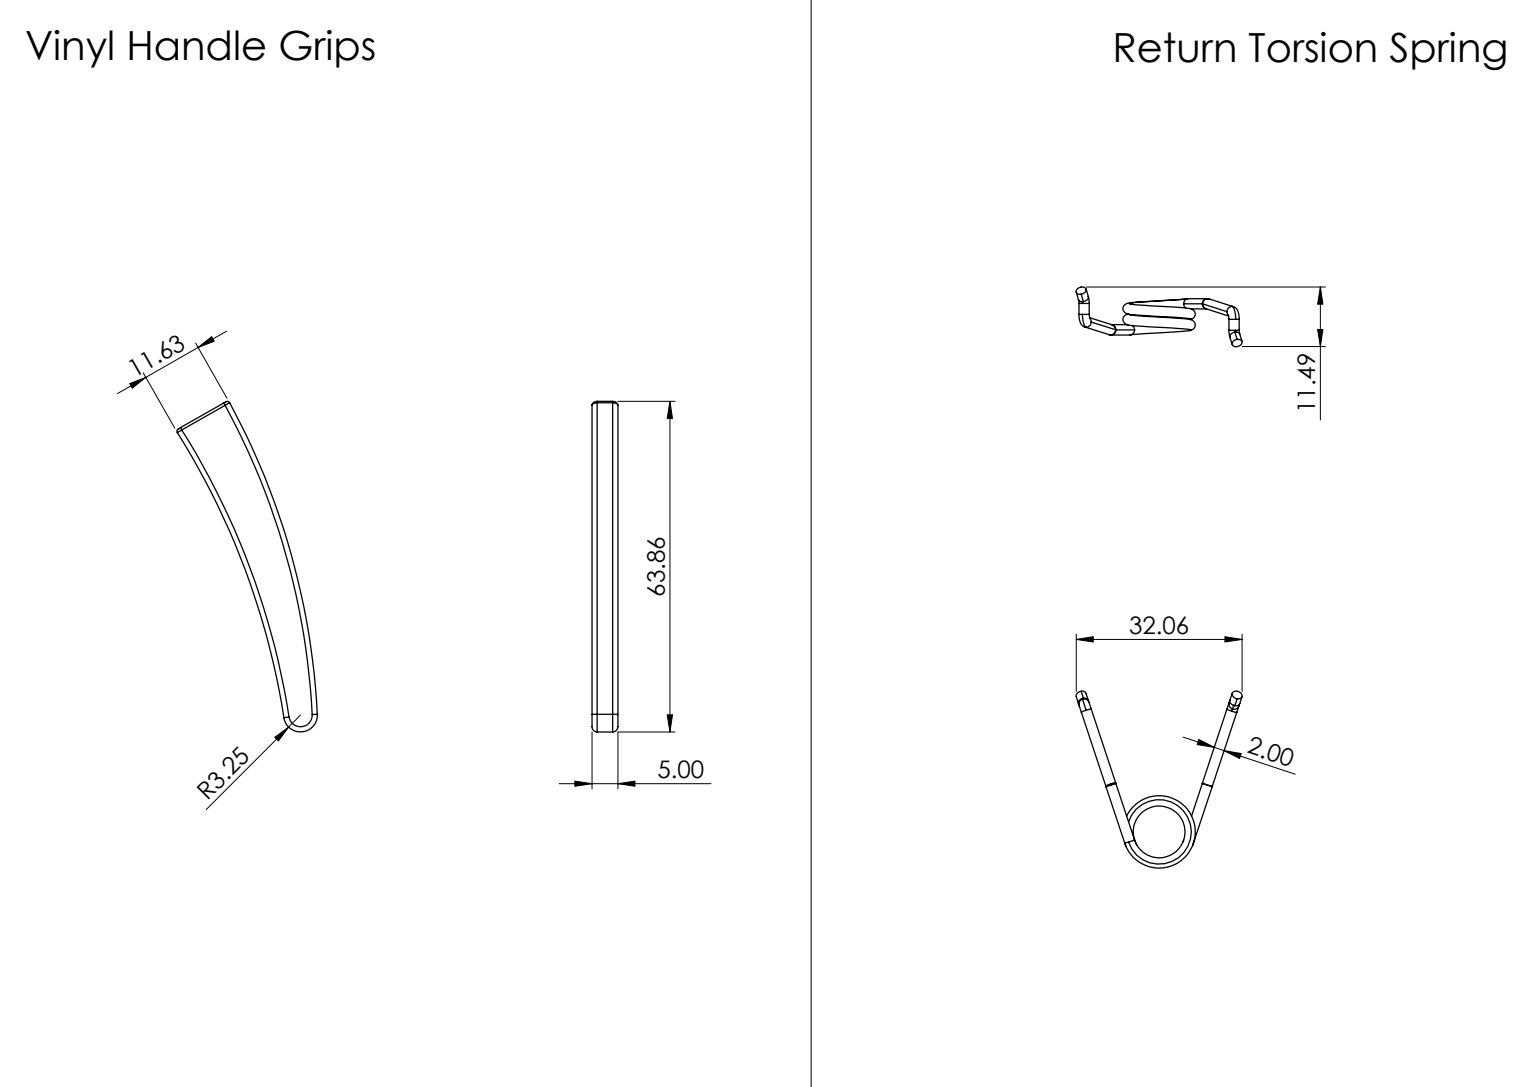
ISO-10303-21;
HEADER;
FILE_DESCRIPTION (('STEP AP214'),
    '1' );
FILE_NAME ('Return Torsion Spring.step',
    '2026-10-09T15:01:35',
    ( '' ),
    ( '' ),
    'SwSTEP 2.0',
    'SolidWorks 2026',
    '' );
FILE_SCHEMA (( 'AUTOMOTIVE_DESIGN' ));
ENDSEC;

DATA;
#6=CARTESIAN_POINT ( 'NONE',  ( -2.243961179877913104, -65.88814609558559710, 1.271710548130833951 ) ) ;
#7=VECTOR ( 'NONE', #4583, 1000.000000000000227 ) ;
#8=CARTESIAN_POINT ( 'NONE',  ( 7.059059989562619819, -58.43975188330606585, -0.3221438859163246460 ) ) ;
#16=CARTESIAN_POINT ( 'NONE',  ( 2.533447467746755333, -55.76293992159236979, -0.1309777151760100067 ) ) ;
#18=FACE_OUTER_BOUND ( 'NONE', #7281, .T. ) ;
#19=CIRCLE ( 'NONE', #5075, 1.000000000000001110 ) ;
#23=LINE ( 'NONE', #5799, #7366 ) ;
#24=AXIS2_PLACEMENT_3D ( 'NONE', #2832, #2306, #6237 ) ;
#29=CARTESIAN_POINT ( 'NONE',  ( -6.272953878096410030, -61.45586155529391448, 1.493064301322690968 ) ) ;
#31=CARTESIAN_POINT ( 'NONE',  ( 1.597826897138040048, -55.24069855439622501, 0.3109211183784004184 ) ) ;
#32=CIRCLE ( 'NONE', #2308, 1.000000000000001110 ) ;
#36=CARTESIAN_POINT ( 'NONE',  ( -15.08175531864075047, -34.71610473016205134, -5.729623873133089518 ) ) ;
#38=EDGE_CURVE ( 'NONE', #489, #1005, #19, .T. ) ;
#39=CARTESIAN_POINT ( 'NONE',  ( 9.311407240687648468, -51.41373841511902043, -1.002481404894999928 ) ) ;
#47=AXIS2_PLACEMENT_3D ( 'NONE', #6946, #1636, #2269 ) ;
#54=CARTESIAN_POINT ( 'NONE',  ( -1.794944750655344867, -54.19869589391355191, -2.224588173883939035 ) ) ;
#57=EDGE_LOOP ( 'NONE', ( #3083, #4276, #3063, #5016, #4331, #6608 ) ) ;
#62=CARTESIAN_POINT ( 'NONE',  ( 3.116905194451685013, -55.41725085606579171, 2.344137946175070653 ) ) ;
#66=ORIENTED_EDGE ( 'NONE', *, *, #4521, .T. ) ;
#67=ORIENTED_EDGE ( 'NONE', *, *, #4872, .T. ) ;
#71=CARTESIAN_POINT ( 'NONE',  ( 1.531562167974070077, -54.12800115838471271, -2.047325108518057935 ) ) ;
#73=CARTESIAN_POINT ( 'NONE',  ( 3.016248221826935083, -64.97666327952782694, -3.135076956698916728 ) ) ;
#78=( NAMED_UNIT ( * ) SI_UNIT ( $, .STERADIAN. ) SOLID_ANGLE_UNIT ( ) );
#80=CARTESIAN_POINT ( 'NONE',  ( 8.409045811045761099, -50.95764513735950629, -2.495037190209991707 ) ) ;
#85=CARTESIAN_POINT ( 'NONE',  ( -4.132930949989339631, -63.16624423302310021, 2.163545901557570428 ) ) ;
#86=DIRECTION ( 'NONE',  ( -0.5224671166576538850, 0.8526594349512809368, 0.000000000000000000 ) ) ;
#87=FACE_OUTER_BOUND ( 'NONE', #3155, .T. ) ;
#94=CARTESIAN_POINT ( 'NONE',  ( -2.961840227416660198, -65.56364223063081909, 1.283932781279834900 ) ) ;
#95=CARTESIAN_POINT ( 'NONE',  ( -1.892846266465454841, -54.28526762408564110, -0.1610563749503846620 ) ) ;
#102=CARTESIAN_POINT ( 'NONE',  ( 2.906897738665179975, -66.25564029441702019, 0.8681355557765302322 ) ) ;
#103=DIRECTION ( 'NONE',  ( 0.2223191033124284066, 0.6712482523644728305, 0.7071067811865467956 ) ) ;
#109=CARTESIAN_POINT ( 'NONE',  ( 5.682346379326408403, -62.38461083188095557, -3.511065069215000278 ) ) ;
#113=CARTESIAN_POINT ( 'NONE',  ( 1.437675307311687245, -54.36893612802973763, 0.01823407963783662405 ) ) ;
#116=CARTESIAN_POINT ( 'NONE',  ( 4.115360779042029904, -63.19255852436059229, -2.695130055691413506 ) ) ;
#121=CARTESIAN_POINT ( 'NONE',  ( 2.653562475325737857, -65.64394347387724338, 0.9832085570212988346 ) ) ;
#123=VERTEX_POINT ( 'NONE', #4619 ) ;
#124=CARTESIAN_POINT ( 'NONE',  ( -5.765066695091211280, -62.35357808832723947, 3.545399627195713332 ) ) ;
#127=CARTESIAN_POINT ( 'NONE',  ( 1.275220786007323914, -54.66846601681689322, 0.1350250863793004130 ) ) ;
#128=CARTESIAN_POINT ( 'NONE',  ( 2.080482015124565098, -66.54183146390657555, -1.221303033644861813 ) ) ;
#129=DIRECTION ( 'NONE',  ( -1.602374898470634869E-16, 1.442524254523139935E-17, 1.000000000000000000 ) ) ;
#135=CARTESIAN_POINT ( 'NONE',  ( -6.814417183322500016, -58.48210382454914935, -0.1019614231452001113 ) ) ;
#144=DIRECTION ( 'NONE',  ( 0.2223157560262044585, -0.6712493609847989262, 0.7071067811865449082 ) ) ;
#146=CIRCLE ( 'NONE', #7235, 1.000000000000000888 ) ;
#149=CARTESIAN_POINT ( 'NONE',  ( -5.163597282883630513, -63.01551968439245144, 3.580859834736030312 ) ) ;
#151=VECTOR ( 'NONE', #4371, 999.9999999999998863 ) ;
#153=CARTESIAN_POINT ( 'NONE',  ( -4.969000869418408683, -63.40403411709974790, -2.714243491562927879 ) ) ;
#154=CARTESIAN_POINT ( 'NONE',  ( -2.104778383727555102, -66.59261038346899397, 1.133408834283370137 ) ) ;
#157=CIRCLE ( 'NONE', #1946, 1.000000000000000444 ) ;
#158=EDGE_LOOP ( 'NONE', ( #2587, #5336, #2767, #4336, #3455, #7221 ) ) ;
#159=PRODUCT_DEFINITION_FORMATION_WITH_SPECIFIED_SOURCE ( 'ANY', '', #255, .NOT_KNOWN. ) ;
#162=EDGE_CURVE ( 'NONE', #6490, #232, #2554, .T. ) ;
#167=CARTESIAN_POINT ( 'NONE',  ( -6.199032880790720235, -61.56120177486793210, 3.556545127952429830 ) ) ;
#170=CARTESIAN_POINT ( 'NONE',  ( 5.465222000274489567, -57.03231251543625291, 0.2812537129946697800 ) ) ;
#177=DIRECTION ( 'NONE',  ( -0.9492883822130750993, 0.3144066910790588865, 0.000000000000000000 ) ) ;
#179=CARTESIAN_POINT ( 'NONE',  ( 5.575556491096470779, -57.10417477796837460, -1.782215851858570010 ) ) ;
#180=CARTESIAN_POINT ( 'NONE',  ( 9.311407240687648468, -51.41373841511900622, -2.502481404895003259 ) ) ;
#188=DIRECTION ( 'NONE',  ( 0.3128416502900965290, -0.9445788350777319931, 0.09950339776592478924 ) ) ;
#189=CARTESIAN_POINT ( 'NONE',  ( -3.569041007005829602, -65.81017109676685095, 3.284668648760890264 ) ) ;
#192=CARTESIAN_POINT ( 'NONE',  ( -2.392055737067099841, -65.19778216667813808, -1.190937291917544050 ) ) ;
#193=CARTESIAN_POINT ( 'NONE',  ( -14.49899450467539985, -35.75040780681265318, -0.4662714048949997969 ) ) ;
#195=CARTESIAN_POINT ( 'NONE',  ( -3.055077159899213690, -65.35589988530520600, -0.7735514844714416194 ) ) ;
#197=CARTESIAN_POINT ( 'NONE',  ( 3.257640280419950241, -66.06664283717124420, -1.252360977842533751 ) ) ;
#203=CARTESIAN_POINT ( 'NONE',  ( -3.235261603508409856, -66.01500717273368934, 1.164464255201294929 ) ) ;
#204=CARTESIAN_POINT ( 'NONE',  ( -5.227302941343250353, -58.92678856866081105, -0.2192372590660296439 ) ) ;
#205=CARTESIAN_POINT ( 'NONE',  ( -6.490403473174280791, -62.28500686936251185, 3.403714661497959870 ) ) ;
#210=VERTEX_POINT ( 'NONE', #2865 ) ;
#214=CARTESIAN_POINT ( 'NONE',  ( 14.18471095241310032, -36.69976849081635351, 0.4975185951050001831 ) ) ;
#215=CARTESIAN_POINT ( 'NONE',  ( -1.756031117750795234, -65.59594772693552045, 1.371125244074580030 ) ) ;
#217=EDGE_CURVE ( 'NONE', #3483, #2618, #2661, .T. ) ;
#224=CARTESIAN_POINT ( 'NONE',  ( -6.308476396955129850, -59.14191327212131455, -0.5142043607924547954 ) ) ;
#226=EDGE_CURVE ( 'NONE', #477, #1089, #6052, .T. ) ;
#228=CARTESIAN_POINT ( 'NONE',  ( -5.725946002089390419, -61.92844332740136792, 1.548851071596535123 ) ) ;
#231=CARTESIAN_POINT ( 'NONE',  ( 2.221695044209367698, -65.89517911169727427, -1.088420971642926727 ) ) ;
#232=VERTEX_POINT ( 'NONE', #3010 ) ;
#239=CARTESIAN_POINT ( 'NONE',  ( -6.429839020462739363, -63.58404662519255623, 2.770540757372710328 ) ) ;
#243=AXIS2_PLACEMENT_3D ( 'NONE', #3684, #2023, #7044 ) ;
#246=CARTESIAN_POINT ( 'NONE',  ( -5.466570931786790766, -63.95713299600960511, -2.842748680216657942 ) ) ;
#247=CARTESIAN_POINT ( 'NONE',  ( 2.831152723192955190, -54.81765481733766876, 0.09675599308719184943 ) ) ;
#255=PRODUCT ( 'Return Torsion Spring', 'Return Torsion Spring', '', ( #964 ) ) ;
#258=CARTESIAN_POINT ( 'NONE',  ( -5.971666637568279867, -56.84728173661435591, 1.574849794282134896 ) ) ;
#262=CARTESIAN_POINT ( 'NONE',  ( 4.897692307440769888, -62.02301377339387756, -1.765793165935516829 ) ) ;
#267=CARTESIAN_POINT ( 'NONE',  ( 3.367951392835606406, -65.15049214652208320, -1.167130348240442927 ) ) ;
#272=DIRECTION ( 'NONE',  ( 0.3128463504745285229, 0.9445772445362839997, 0.09950371902099811039 ) ) ;
#276=CARTESIAN_POINT ( 'NONE',  ( -3.156642594714314853, -54.82761582543010093, 1.871643660998590697 ) ) ;
#278=CARTESIAN_POINT ( 'NONE',  ( -1.626396133375414887, -53.66552156771879112, 1.839959185157149957 ) ) ;
#279=DIRECTION ( 'NONE',  ( 0.000000000000000000, -0.7252570966694442678, 0.6884781359858920258 ) ) ;
#289=CARTESIAN_POINT ( 'NONE',  ( 1.662636012147085118, -65.62619303409478277, -3.045852711070930141 ) ) ;
#290=CARTESIAN_POINT ( 'NONE',  ( 4.774359225188401723, -64.47360709931102463, 0.6998940494460414996 ) ) ;
#292=ORIENTED_EDGE ( 'NONE', *, *, #6726, .T. ) ;
#295=ORIENTED_EDGE ( 'NONE', *, *, #5689, .F. ) ;
#296=DIRECTION ( 'NONE',  ( 0.9492899500389736511, 0.3144019573014823488, 0.000000000000000000 ) ) ;
#300=CARTESIAN_POINT ( 'NONE',  ( 6.696612653858620590, -58.50870383553881737, 0.2496331057155200817 ) ) ;
#303=EDGE_CURVE ( 'NONE', #4768, #4244, #4606, .T. ) ;
#306=CARTESIAN_POINT ( 'NONE',  ( -5.408997660349871062, -62.29959681528816873, 3.625047998704080232 ) ) ;
#309=CARTESIAN_POINT ( 'NONE',  ( -0.5318364440386327274, -66.20751837745356738, -3.028967907328838027 ) ) ;
#311=ORIENTED_EDGE ( 'NONE', *, *, #217, .T. ) ;
#312=CARTESIAN_POINT ( 'NONE',  ( 14.02750760687355935, -37.17441268192290238, 0.4975185951050001831 ) ) ;
#314=DIRECTION ( 'NONE',  ( 0.3128416502900965290, -0.9445788350777319931, 0.09950339776592478924 ) ) ;
#315=DIRECTION ( 'NONE',  ( -0.4328040977884316520, 0.5819352847797604200, 0.6884997728872834788 ) ) ;
#317=CARTESIAN_POINT ( 'NONE',  ( 6.075450823322679383, -63.85990335785957228, 0.5148622082158803570 ) ) ;
#324=CARTESIAN_POINT ( 'NONE',  ( -4.747117373927349782, -63.10583374278928659, -0.4844647803776696016 ) ) ;
#326=CARTESIAN_POINT ( 'NONE',  ( -4.385465831998347497, -64.89496069624793506, 1.250664309176121813 ) ) ;
#327=VERTEX_POINT ( 'NONE', #3117 ) ;
#335=CARTESIAN_POINT ( 'NONE',  ( 1.944327905822930136, -53.75057748617523856, 2.017748614706070143 ) ) ;
#336=ORIENTED_EDGE ( 'NONE', *, *, #6986, .T. ) ;
#338=CARTESIAN_POINT ( 'NONE',  ( -1.512046953658800152, -54.18079592905042574, 1.959428465566195543 ) ) ;
#339=EDGE_CURVE ( 'NONE', #4174, #2620, #4361, .T. ) ;
#350=CARTESIAN_POINT ( 'NONE',  ( 3.592758869166885471, -66.41582265024271692, 0.6922273147611399668 ) ) ;
#354=VERTEX_POINT ( 'NONE', #1399 ) ;
#359=CARTESIAN_POINT ( 'NONE',  ( -5.294444503516980483, -61.70453834742492916, -0.3952116983248150084 ) ) ;
#361=CARTESIAN_POINT ( 'NONE',  ( -6.248181790555211279, -60.49255085186674563, 1.512929826500920338 ) ) ;
#362=CARTESIAN_POINT ( 'NONE',  ( -4.797760869400969241, -62.71499483963494015, 1.636667228454699696 ) ) ;
#367=( NAMED_UNIT ( * ) PLANE_ANGLE_UNIT ( ) SI_UNIT ( $, .RADIAN. ) );
#371=CARTESIAN_POINT ( 'NONE',  ( 6.135463341229070444, -63.36916140199613778, -1.604994752452352014 ) ) ;
#374=ADVANCED_FACE ( 'NONE', ( #1915 ), #2901, .T. ) ;
#377=CARTESIAN_POINT ( 'NONE',  ( 15.08188723176695056, -33.99092340910145538, 5.072392329257909616 ) ) ;
#378=DIRECTION ( 'NONE',  ( 0.000000000000000000, -0.7252570966694443788, 0.6884781359858918037 ) ) ;
#380=VERTEX_POINT ( 'NONE', #6559 ) ;
#382=B_SPLINE_CURVE_WITH_KNOTS ( 'NONE', 3,
 ( #5287, #6445, #2450, #5362, #4685, #5889 ),
 .UNSPECIFIED., .F., .F.,
 ( 4, 2, 4 ),
 ( 0.000000000000000000, 0.5000000000000000000, 1.000000000000000000 ),
 .UNSPECIFIED. ) ;
#388=CARTESIAN_POINT ( 'NONE',  ( -6.381106047699259598, -62.60757382768967716, 3.386766328596300113 ) ) ;
#390=AXIS2_PLACEMENT_3D ( 'NONE', #1613, #3079, #7288 ) ;
#396=CARTESIAN_POINT ( 'NONE',  ( 14.63724902514210058, -34.60816281716094522, 2.969700630898919780 ) ) ;
#400=CARTESIAN_POINT ( 'NONE',  ( -4.470547512179178895, -58.04376326654274720, -1.678768375691622960 ) ) ;
#402=CARTESIAN_POINT ( 'NONE',  ( -4.067320158550557174, -55.70390554630877489, -0.2964418605464455014 ) ) ;
#408=CIRCLE ( 'NONE', #6306, 1.000000000000000888 ) ;
#414=CARTESIAN_POINT ( 'NONE',  ( -3.723298236168965047, -66.76642012610518861, 0.4732191326009700938 ) ) ;
#424=AXIS2_PLACEMENT_3D ( 'NONE', #4211, #6401, #703 ) ;
#425=FACE_OUTER_BOUND ( 'NONE', #7112, .T. ) ;
#426=CARTESIAN_POINT ( 'NONE',  ( -6.269521507055145548, -62.51903585589134593, 1.741451463471350936 ) ) ;
#432=CARTESIAN_POINT ( 'NONE',  ( -1.862703854971429873, -67.54117654042293850, 0.3860096597272351659 ) ) ;
#436=CARTESIAN_POINT ( 'NONE',  ( -2.708443266796834781, -56.15294253968003346, -1.503436295530243827 ) ) ;
#440=EDGE_CURVE ( 'NONE', #477, #6355, #744, .T. ) ;
#441=CARTESIAN_POINT ( 'NONE',  ( 1.159677199572074269, -55.50330010691895666, -1.238196965061255650 ) ) ;
#454=CARTESIAN_POINT ( 'NONE',  ( 1.349182120017575981, -67.40498645023109248, 1.310568389067595207 ) ) ;
#455=DIRECTION ( 'NONE',  ( -0.4328040977884316520, 0.5819352847797604200, 0.6884997728872834788 ) ) ;
#458=LINE ( 'NONE', #3308, #1211 ) ;
#459=CARTESIAN_POINT ( 'NONE',  ( -6.392983792945144295, -62.56006988191466434, 1.848553975009203487 ) ) ;
#465=CARTESIAN_POINT ( 'NONE',  ( 6.751207790105429929, -62.61097121624884210, 0.9581327554396804613 ) ) ;
#469=ADVANCED_FACE ( 'NONE', ( #5653 ), #6728, .T. ) ;
#470=CARTESIAN_POINT ( 'NONE',  ( -1.128062821581302000, -55.49617455686423284, 0.7066123397475153611 ) ) ;
#473=CARTESIAN_POINT ( 'NONE',  ( 1.277257345132870148, -65.35512402512885899, -0.3535023904437397113 ) ) ;
#475=CARTESIAN_POINT ( 'NONE',  ( 4.746441911065370611, -62.01614811949030326, -2.502481404895003259 ) ) ;
#476=CARTESIAN_POINT ( 'NONE',  ( -3.427937952159080037, -54.92350006295870202, -2.312565912944844371 ) ) ;
#477=VERTEX_POINT ( 'NONE', #6809 ) ;
#480=AXIS2_PLACEMENT_3D ( 'NONE', #1466, #4941, #1989 ) ;
#482=EDGE_LOOP ( 'NONE', ( #4891, #695, #2259, #4148, #2799, #2578 ) ) ;
#486=CARTESIAN_POINT ( 'NONE',  ( 3.523276076382420019, -54.00647132653568860, -0.5873174244349146367 ) ) ;
#489=VERTEX_POINT ( 'NONE', #4526 ) ;
#492=CARTESIAN_POINT ( 'NONE',  ( -9.311346830843399758, -51.41373841511900622, 2.533728595105000370 ) ) ;
#493=ADVANCED_FACE ( 'NONE', ( #6254 ), #1091, .T. ) ;
#495=CARTESIAN_POINT ( 'NONE',  ( -5.206993624623629913, -63.95781028998001716, 3.417603084305509853 ) ) ;
#500=CIRCLE ( 'NONE', #2164, 0.9999999999999986677 ) ;
#501=ORIENTED_EDGE ( 'NONE', *, *, #5222, .F. ) ;
#503=CARTESIAN_POINT ( 'NONE',  ( -4.748090069711009775, -62.01667038360579198, 2.533819555318849837 ) ) ;
#505=CARTESIAN_POINT ( 'NONE',  ( -1.424128410011220147, -67.64226375110297340, -1.734372748508781870 ) ) ;
#508=ORIENTED_EDGE ( 'NONE', *, *, #1767, .F. ) ;
#509=CARTESIAN_POINT ( 'NONE',  ( -4.739687333205909958, -61.73825078254577647, 2.268939929871689909 ) ) ;
#510=CARTESIAN_POINT ( 'NONE',  ( 8.362118858474568484, -51.09933172403994917, -2.502481404895003259 ) ) ;
#511=LINE ( 'NONE', #5719, #6770 ) ;
#513=CARTESIAN_POINT ( 'NONE',  ( -5.135436550704829628, -59.04801135763068487, 1.370314102932454814 ) ) ;
#517=CARTESIAN_POINT ( 'NONE',  ( -5.091256589979570535, -61.80182140578926919, 1.697438579844070761 ) ) ;
#519=ORIENTED_EDGE ( 'NONE', *, *, #2113, .F. ) ;
#520=AXIS2_PLACEMENT_3D ( 'NONE', #4684, #6372, #4184 ) ;
#522=CIRCLE ( 'NONE', #1723, 0.9999999999999998890 ) ;
#523=CARTESIAN_POINT ( 'NONE',  ( -13.12502771320784056, -36.71825441132875767, 1.026284428608169819 ) ) ;
#525=CARTESIAN_POINT ( 'NONE',  ( -7.069128816957480410, -61.66762450778810489, 2.866206824378770168 ) ) ;
#538=ORIENTED_EDGE ( 'NONE', *, *, #4985, .F. ) ;
#539=TOROIDAL_SURFACE ( 'NONE', #424, 1.500000000000000000, 1.000000000000000000 ) ;
#544=CARTESIAN_POINT ( 'NONE',  ( 3.523276076382420019, -54.00647132653568860, -0.5873174244349146367 ) ) ;
#545=CARTESIAN_POINT ( 'NONE',  ( -6.643389330756649613, -62.64438243220202196, 2.533637634891150459 ) ) ;
#547=CARTESIAN_POINT ( 'NONE',  ( -4.835761215296770388, -62.04624743670729003, 2.958213919140463055 ) ) ;
#550=CARTESIAN_POINT ( 'NONE',  ( 4.922451174039159660, -61.67826628571419434, -0.7081498598146799273 ) ) ;
#562=CARTESIAN_POINT ( 'NONE',  ( -1.564844514157090138, -53.52797147715784121, 0.2502733031487548443 ) ) ;
#570=ORIENTED_EDGE ( 'NONE', *, *, #4038, .F. ) ;
#571=B_SPLINE_CURVE_WITH_KNOTS ( 'NONE', 3,
 ( #1251, #3568, #5855, #6893, #2994, #3601, #5309, #109, #4035, #643 ),
 .UNSPECIFIED., .F., .F.,
 ( 4, 2, 2, 2, 4 ),
 ( 0.000000000000000000, 0.2500000000000000000, 0.5000000000000000000, 0.7500000000000000000, 1.000000000000000000 ),
 .UNSPECIFIED. ) ;
#574=CARTESIAN_POINT ( 'NONE',  ( -5.480856739662490540, -62.25220485324549458, 1.560007870815685260 ) ) ;
#575=CARTESIAN_POINT ( 'NONE',  ( -1.985532163257450078, -53.63691243282757881, -1.870211432998861945 ) ) ;
#583=CARTESIAN_POINT ( 'NONE',  ( -2.642495264810874822, -65.73545435749777255, -0.8365618114303696728 ) ) ;
#589=CARTESIAN_POINT ( 'NONE',  ( -15.08175531864075047, -33.99084820126180517, -5.041145139047909396 ) ) ;
#591=CARTESIAN_POINT ( 'NONE',  ( -6.240992105565960735, -57.07993508854151798, -2.135104940435555765 ) ) ;
#593=CARTESIAN_POINT ( 'NONE',  ( 5.330483863435800274, -59.34891080545844488, 0.6651839376153853012 ) ) ;
#594=EDGE_LOOP ( 'NONE', ( #6937, #821, #6883, #4560, #734, #2839 ) ) ;
#597=DIRECTION ( 'NONE',  ( -0.08966155106958693943, -0.9959722919136836383, 0.000000000000000000 ) ) ;
#607=DIRECTION ( 'NONE',  ( 0.2223191033124283789, 0.6712482523644727195, 0.7071067811865466846 ) ) ;
#608=CARTESIAN_POINT ( 'NONE',  ( 3.189415849367489564, -54.78201482374456788, -1.959602550130806753 ) ) ;
#616=CARTESIAN_POINT ( 'NONE',  ( -14.63712380658832046, -34.60809039433110001, -2.938452842589635683 ) ) ;
#617=CARTESIAN_POINT ( 'NONE',  ( 5.661089107917369745, -62.15448909529578003, 2.785446686898291002 ) ) ;
#628=AXIS2_PLACEMENT_3D ( 'NONE', #5622, #2168, #455 ) ;
#630=CARTESIAN_POINT ( 'NONE',  ( 1.773380156858839873, -67.30899524596459571, -0.8098396333890448551 ) ) ;
#632=CARTESIAN_POINT ( 'NONE',  ( 2.959376181595404720, -55.87711464508088710, 0.4000749283577051951 ) ) ;
#635=ORIENTED_EDGE ( 'NONE', *, *, #339, .F. ) ;
#636=CIRCLE ( 'NONE', #748, 0.9999999999999984457 ) ;
#643=CARTESIAN_POINT ( 'NONE',  ( 5.463696144088109996, -62.30361170774578028, -3.475027489484119769 ) ) ;
#644=CARTESIAN_POINT ( 'NONE',  ( -5.563801105733269914, -63.69014839564722763, 1.341242183458755344 ) ) ;
#645=CARTESIAN_POINT ( 'NONE',  ( 14.41492992182968003, -36.00466816619485400, 4.365285548071359045 ) ) ;
#648=CARTESIAN_POINT ( 'NONE',  ( 2.466033592522905327, -56.00841680802438560, -1.148886392136307943 ) ) ;
#651=CARTESIAN_POINT ( 'NONE',  ( 14.10571919449219891, -36.93826837078879777, -1.990074380419982969 ) ) ;
#653=CARTESIAN_POINT ( 'NONE',  ( 5.771550998859873438, -61.36048738820532122, 0.6685664931038850511 ) ) ;
#654=CARTESIAN_POINT ( 'NONE',  ( 1.915558458284230214, -54.23376817553720031, 0.07315972318039029587 ) ) ;
#658=CARTESIAN_POINT ( 'NONE',  ( -5.343639688141238686, -62.21333143151184686, 3.460348891136710403 ) ) ;
#662=CARTESIAN_POINT ( 'NONE',  ( 1.919155946380425082, -66.03927477571377835, -1.101811511879709826 ) ) ;
#663=CARTESIAN_POINT ( 'NONE',  ( -2.887726905928315269, -66.20272978495717098, -0.9560320787877147897 ) ) ;
#669=EDGE_CURVE ( 'NONE', #3171, #6921, #5083, .T. ) ;
#672=CARTESIAN_POINT ( 'NONE',  ( -3.268733238405740149, -66.73531384189965365, -2.665188268689791862 ) ) ;
#681=CARTESIAN_POINT ( 'NONE',  ( 5.090297305459900556, -61.99464686763499088, 2.430409751936420282 ) ) ;
#683=CARTESIAN_POINT ( 'NONE',  ( 14.97072768011073940, -34.32654753528365177, 2.597518595105000383 ) ) ;
#685=CARTESIAN_POINT ( 'NONE',  ( 6.202282335592980367, -63.50128988325390367, -3.194577187992014622 ) ) ;
#690=CARTESIAN_POINT ( 'NONE',  ( -5.250750166908019878, -57.72135505925717069, -0.3064819419056146188 ) ) ;
#691=CARTESIAN_POINT ( 'NONE',  ( 1.316624512147740012, -66.75104842734066324, 3.019790780136459851 ) ) ;
#692=CARTESIAN_POINT ( 'NONE',  ( 14.49911764349215915, -35.75048010860329839, 0.4975185951050001831 ) ) ;
#693=ORIENTED_EDGE ( 'NONE', *, *, #5607, .F. ) ;
#695=ORIENTED_EDGE ( 'NONE', *, *, #4767, .T. ) ;
#699=CARTESIAN_POINT ( 'NONE',  ( -6.321361399357500410, -61.94876894069515316, -0.6341497168666246909 ) ) ;
#701=ORIENTED_EDGE ( 'NONE', *, *, #1180, .T. ) ;
#703=DIRECTION ( 'NONE',  ( 0.3144019573014849023, -0.9492899500389726519, 0.000000000000000000 ) ) ;
#705=CARTESIAN_POINT ( 'NONE',  ( -1.512046953658800152, -54.18079592905042574, 1.959428465566195543 ) ) ;
#707=EDGE_CURVE ( 'NONE', #3483, #3171, #4003, .T. ) ;
#708=CARTESIAN_POINT ( 'NONE',  ( -2.678905510920184696, -65.04233304593640241, 0.9295552878624004922 ) ) ;
#711=CARTESIAN_POINT ( 'NONE',  ( 14.49911764349215915, -35.75048010860329839, 0.4975185951050001831 ) ) ;
#712=CARTESIAN_POINT ( 'NONE',  ( -0.07696283880832878455, -66.23396610719073863, -3.055188877874750020 ) ) ;
#713=CARTESIAN_POINT ( 'NONE',  ( -5.316774007586650086, -63.89131393482077925, 1.354123676545745170 ) ) ;
#715=CIRCLE ( 'NONE', #1687, 1.000000000000000444 ) ;
#723=CARTESIAN_POINT ( 'NONE',  ( 1.159215146223531834, -55.24985087088717250, -0.2200125624336850272 ) ) ;
#724=CARTESIAN_POINT ( 'NONE',  ( -6.708998324124310741, -61.63987295270813860, 3.437611327301279385 ) ) ;
#732=CARTESIAN_POINT ( 'NONE',  ( -1.855492712959899926, -67.28785520969887557, -0.6321745227666250022 ) ) ;
#734=ORIENTED_EDGE ( 'NONE', *, *, #3822, .F. ) ;
#737=CARTESIAN_POINT ( 'NONE',  ( -14.81339646197689852, -34.80111785677370051, -2.566271404894997499 ) ) ;
#738=EDGE_CURVE ( 'NONE', #7318, #1826, #636, .T. ) ;
#739=DIRECTION ( 'NONE',  ( 0.3144066910790611624, 0.9492883822130743221, 0.000000000000000000 ) ) ;
#743=AXIS2_PLACEMENT_3D ( 'NONE', #312, #6591, #3835 ) ;
#744=CIRCLE ( 'NONE', #628, 1.000000000000000888 ) ;
#747=CARTESIAN_POINT ( 'NONE',  ( 1.626596344682255113, -54.75750786503496670, 2.255510009909589719 ) ) ;
#748=AXIS2_PLACEMENT_3D ( 'NONE', #2153, #1638, #3968 ) ;
#751=AXIS2_PLACEMENT_3D ( 'NONE', #5959, #3597, #6467 ) ;
#753=CARTESIAN_POINT ( 'NONE',  ( -5.431783234843397423, -58.17252153501718226, -0.3016490821137323142 ) ) ;
#754=CARTESIAN_POINT ( 'NONE',  ( 6.180415987647270626, -62.45112898858806716, 0.6030958204723052551 ) ) ;
#756=ORIENTED_EDGE ( 'NONE', *, *, #1602, .T. ) ;
#764=CARTESIAN_POINT ( 'NONE',  ( -6.097705871868670080, -61.85866295707492668, 3.539665806518350610 ) ) ;
#766=CARTESIAN_POINT ( 'NONE',  ( -2.527830428429834964, -65.26309079616396502, -2.780623214462280668 ) ) ;
#768=CARTESIAN_POINT ( 'NONE',  ( -6.129265975028279634, -62.42766041111902098, -0.6909925287373350766 ) ) ;
#773=ORIENTED_EDGE ( 'NONE', *, *, #2365, .T. ) ;
#777=CARTESIAN_POINT ( 'NONE',  ( 5.248671903609490208, -63.99330799355751509, -3.505550301244489741 ) ) ;
#780=DIRECTION ( 'NONE',  ( 0.2164621326156030423, -0.07169280077033016174, 0.9736551173085935540 ) ) ;
#783=CARTESIAN_POINT ( 'NONE',  ( -6.097705871868670080, -61.85866295707492668, 3.539665806518350610 ) ) ;
#784=ORIENTED_EDGE ( 'NONE', *, *, #6468, .F. ) ;
#785=EDGE_LOOP ( 'NONE', ( #5644, #3488, #7009, #2675, #2047, #4651 ) ) ;
#788=CARTESIAN_POINT ( 'NONE',  ( 4.977719985769329725, -63.63849604921595216, 2.874328699340139792 ) ) ;
#789=CARTESIAN_POINT ( 'NONE',  ( 9.311407240687648468, -51.41373841511902043, -1.002481404894999928 ) ) ;
#791=CARTESIAN_POINT ( 'NONE',  ( 4.372548960228861858, -64.23807538291029573, -1.245661913065559734 ) ) ;
#798=CARTESIAN_POINT ( 'NONE',  ( 5.661113010068490325, -57.37064013373739613, 2.401523511004880262 ) ) ;
#799=FACE_OUTER_BOUND ( 'NONE', #1045, .T. ) ;
#801=ORIENTED_EDGE ( 'NONE', *, *, #2322, .T. ) ;
#805=CARTESIAN_POINT ( 'NONE',  ( 9.358334193258830425, -51.27205182843857045, -2.495037190209991707 ) ) ;
#806=DIRECTION ( 'NONE',  ( -0.3144066910790599412, -0.9492883822130747662, 0.000000000000000000 ) ) ;
#807=CARTESIAN_POINT ( 'NONE',  ( 2.440761905804889942, -65.30842328614467363, 1.105894752426585415 ) ) ;
#808=CARTESIAN_POINT ( 'NONE',  ( -5.904042796847299712, -62.42803713013675093, 3.506543003539000392 ) ) ;
#817=CARTESIAN_POINT ( 'NONE',  ( -0.9970853242166300978, -65.67144495878099519, -1.280490079922569802 ) ) ;
#820=CARTESIAN_POINT ( 'NONE',  ( 4.754243898017194603, -57.04914850836969009, -1.691473023288849742 ) ) ;
#821=ORIENTED_EDGE ( 'NONE', *, *, #4240, .T. ) ;
#825=DIRECTION ( 'NONE',  ( 0.1860016876085203719, -0.1636620475539280195, 0.9688230521603200529 ) ) ;
#828=CARTESIAN_POINT ( 'NONE',  ( -1.974098099753330171, -66.57628266072889289, 3.196874607719439876 ) ) ;
#829=CARTESIAN_POINT ( 'NONE',  ( -3.508682979600159957, -66.46637211483655960, 1.044995729122755179 ) ) ;
#833=AXIS2_PLACEMENT_3D ( 'NONE', #2348, #5745, #4043 ) ;
#834=CARTESIAN_POINT ( 'NONE',  ( 9.311407240687648468, -51.41373841511902043, -3.502481404894999706 ) ) ;
#838=CARTESIAN_POINT ( 'NONE',  ( 5.253257825778660184, -59.02147093648149223, -1.455491405082765866 ) ) ;
#839=CARTESIAN_POINT ( 'NONE',  ( 6.214916356356757099, -59.39665835591213749, 2.509282487442340948 ) ) ;
#850=CARTESIAN_POINT ( 'NONE',  ( 3.592758869166885471, -66.41582265024271692, 0.6922273147611399668 ) ) ;
#854=CARTESIAN_POINT ( 'NONE',  ( 14.63724902514210058, -36.05867701049984930, 4.346656902870709160 ) ) ;
#855=CARTESIAN_POINT ( 'NONE',  ( 5.175864525269250116, -61.68163375030346174, 0.3100344153189201202 ) ) ;
#861=CARTESIAN_POINT ( 'NONE',  ( -3.816438721764812136, -64.79865757078124489, -2.819062171272241901 ) ) ;
#865=AXIS2_PLACEMENT_3D ( 'NONE', #7223, #2593, #904 ) ;
#866=CARTESIAN_POINT ( 'NONE',  ( -14.49899450467539985, -35.75040780681265318, -2.566271404894997499 ) ) ;
#870=CARTESIAN_POINT ( 'NONE',  ( -5.628700163094269016, -63.23550210468251009, 3.461537593744290042 ) ) ;
#873=CARTESIAN_POINT ( 'NONE',  ( 6.131131505788760094, -57.13037711201883440, 2.282642250695309905 ) ) ;
#879=ADVANCED_FACE ( 'NONE', ( #799 ), #2886, .T. ) ;
#880=AXIS2_PLACEMENT_3D ( 'NONE', #4624, #4579, #3475 ) ;
#885=CARTESIAN_POINT ( 'NONE',  ( 4.826828241146579934, -57.92957641372471755, 0.5758163846279100717 ) ) ;
#887=CARTESIAN_POINT ( 'NONE',  ( -5.586110484983932700, -63.35381962756557783, 1.355548068171432252 ) ) ;
#898=CARTESIAN_POINT ( 'NONE',  ( 5.267626090836840191, -63.86700364562991439, -1.442031773567929775 ) ) ;
#903=ADVANCED_FACE ( 'NONE', ( #1173 ), #6519, .T. ) ;
#904=DIRECTION ( 'NONE',  ( -0.2163384215910431896, -0.07165063022625259292, 0.9736857165079894072 ) ) ;
#905=CARTESIAN_POINT ( 'NONE',  ( -3.569041007005829602, -65.81017109676685095, 3.284668648760890264 ) ) ;
#906=ORIENTED_EDGE ( 'NONE', *, *, #7286, .F. ) ;
#907=CARTESIAN_POINT ( 'NONE',  ( -6.643389330756649613, -62.64438243220202196, 2.533637634891150459 ) ) ;
#914=CARTESIAN_POINT ( 'NONE',  ( 5.416018991692120643, -63.93240027730202968, 2.754852738177090643 ) ) ;
#915=CARTESIAN_POINT ( 'NONE',  ( 6.647873823884112632, -62.63640551056316497, -2.279271695592409497 ) ) ;
#916=CARTESIAN_POINT ( 'NONE',  ( 6.663059173928499668, -62.48704134639812935, 2.547684199221960100 ) ) ;
#923=CARTESIAN_POINT ( 'NONE',  ( 4.756074659365879143, -62.80135681555328375, -3.311393743080873975 ) ) ;
#926=CARTESIAN_POINT ( 'NONE',  ( -5.894573565049844532, -58.07158296836707478, 1.644009501509583027 ) ) ;
#934=CARTESIAN_POINT ( 'NONE',  ( -1.206827191127304078, -66.77204028133226643, -1.044217440639481742 ) ) ;
#940=CARTESIAN_POINT ( 'NONE',  ( -1.095027572700850049, -66.25608112803911354, -0.9253912358714898589 ) ) ;
#943=EDGE_CURVE ( 'NONE', #2698, #3646, #2185, .T. ) ;
#944=CARTESIAN_POINT ( 'NONE',  ( -5.667613743078470101, -62.32074054030601928, 1.527775587545428193 ) ) ;
#946=CARTESIAN_POINT ( 'NONE',  ( 9.358334193258830425, -51.27205182843857045, -2.495037190209989930 ) ) ;
#948=CARTESIAN_POINT ( 'NONE',  ( 6.319659661046010513, -62.49917928162491876, -1.706589513406323366 ) ) ;
#949=CARTESIAN_POINT ( 'NONE',  ( -1.678659834933539985, -53.30027862203323252, 1.268182062803870247 ) ) ;
#954=CARTESIAN_POINT ( 'NONE',  ( 13.49911764349216092, -35.75048010860329839, 0.4975185951050001831 ) ) ;
#957=CARTESIAN_POINT ( 'NONE',  ( -4.248468832057555211, -63.21868707083201855, -2.033638508047526550 ) ) ;
#959=CARTESIAN_POINT ( 'NONE',  ( 6.164870568366772829, -59.43741054342344654, 0.4113734782956702252 ) ) ;
#964=PRODUCT_CONTEXT ( 'NONE', #2544, 'mechanical' ) ;
#969=CARTESIAN_POINT ( 'NONE',  ( -6.490403473174280791, -62.28500686936251185, 3.403714661497959870 ) ) ;
#973=CARTESIAN_POINT ( 'NONE',  ( 6.285636693253979779, -59.03245517747429716, 2.489777307435960374 ) ) ;
#977=ORIENTED_EDGE ( 'NONE', *, *, #5252, .T. ) ;
#982=LINE ( 'NONE', #1590, #1137 ) ;
#983=DIRECTION ( 'NONE',  ( -0.9492899500389727629, -0.3144019573014849023, 0.000000000000000000 ) ) ;
#984=CARTESIAN_POINT ( 'NONE',  ( 1.349182120017575981, -67.40498645023109248, 1.310568389067595207 ) ) ;
#985=DIRECTION ( 'NONE',  ( 0.1860016876085203441, -0.1636620475539279917, 0.9688230521603200529 ) ) ;
#986=CIRCLE ( 'NONE', #390, 0.9999999999999998890 ) ;
#994=VECTOR ( 'NONE', #5299, 1000.000000000000114 ) ;
#995=DIRECTION ( 'NONE',  ( 0.3144066910790613845, 0.9492883822130742111, 0.000000000000000000 ) ) ;
#996=CARTESIAN_POINT ( 'NONE',  ( -1.630661209647960019, -65.50972637651682362, 2.960670344429949807 ) ) ;
#999=CARTESIAN_POINT ( 'NONE',  ( -4.429163702585058537, -56.03682623248362660, -0.3226722266289872576 ) ) ;
#1001=CARTESIAN_POINT ( 'NONE',  ( 5.674632694949170109, -63.26545500802649258, -3.549449971387770297 ) ) ;
#1005=VERTEX_POINT ( 'NONE', #3490 ) ;
#1010=DIRECTION ( 'NONE',  ( 0.3144066910790610514, 0.9492883822130744331, 0.000000000000000000 ) ) ;
#1013=CARTESIAN_POINT ( 'NONE',  ( -6.126235009943979293, -64.48141016635396738, -1.469515951087519978 ) ) ;
#1018=DIRECTION ( 'NONE',  ( 0.3144019573014853464, -0.9492899500389726519, -7.355227538141627568E-16 ) ) ;
#1019=CARTESIAN_POINT ( 'NONE',  ( 5.929218414971320072, -62.35084102844776055, -1.530333388185332932 ) ) ;
#1028=DIRECTION ( 'NONE',  ( 0.2223157560262043198, -0.6712493609847984821, 0.7071067811865453523 ) ) ;
#1030=CARTESIAN_POINT ( 'NONE',  ( 4.128395891713080523, -66.51223636356003510, -1.999098658498605019 ) ) ;
#1033=VERTEX_POINT ( 'NONE', #36 ) ;
#1035=CARTESIAN_POINT ( 'NONE',  ( -4.410792138572509735, -62.95272468751611683, 0.08690264739508006542 ) ) ;
#1038=CARTESIAN_POINT ( 'NONE',  ( -4.317466541193835106, -57.77653723152862142, 0.4415034884863752729 ) ) ;
#1041=CARTESIAN_POINT ( 'NONE',  ( -0.4891006619385195320, -66.67017596358577691, -1.083201131225852265 ) ) ;
#1043=EDGE_CURVE ( 'NONE', #1750, #4040, #3536, .T. ) ;
#1045=EDGE_LOOP ( 'NONE', ( #4028, #1415, #2287, #784, #2380, #4918 ) ) ;
#1049=DIRECTION ( 'NONE',  ( -1.602374898470634869E-16, 1.442524254523139935E-17, 1.000000000000000000 ) ) ;
#1051=CARTESIAN_POINT ( 'NONE',  ( -5.957512881900739465, -64.40555820178136059, 2.727170671215090270 ) ) ;
#1057=CARTESIAN_POINT ( 'NONE',  ( -6.308476396955129850, -59.14191327212131455, -0.5142043607924547954 ) ) ;
#1066=CARTESIAN_POINT ( 'NONE',  ( 7.124841322228030904, -62.19900605811294980, -0.1440571144897197509 ) ) ;
#1070=CARTESIAN_POINT ( 'NONE',  ( 4.447965418036755381, -62.61493371638615457, -2.739923498411994451 ) ) ;
#1075=CARTESIAN_POINT ( 'NONE',  ( -9.358272925367041140, -51.27205205187813419, 2.526284428608170263 ) ) ;
#1076=CARTESIAN_POINT ( 'NONE',  ( -5.318175601589866908, -63.71090186687732171, -0.7685412544916830901 ) ) ;
#1077=CARTESIAN_POINT ( 'NONE',  ( -6.338727533122220592, -59.01378846946391832, -2.577673957235475211 ) ) ;
#1080=ORIENTED_EDGE ( 'NONE', *, *, #1641, .T. ) ;
#1088=CARTESIAN_POINT ( 'NONE',  ( -3.941959611298590183, -54.25574829393653431, -0.9393447306324897994 ) ) ;
#1089=VERTEX_POINT ( 'NONE', #737 ) ;
#1091=CYLINDRICAL_SURFACE ( 'NONE', #6752, 0.9999999999999988898 ) ;
#1100=CIRCLE ( 'NONE', #3980, 0.9999999999999986677 ) ;
#1104=CARTESIAN_POINT ( 'NONE',  ( -15.08175531864075047, -33.26559167236155190, -4.352666404962730162 ) ) ;
#1105=CARTESIAN_POINT ( 'NONE',  ( -6.238287558858839787, -63.42668406018486849, 1.752565146537014895 ) ) ;
#1108=CARTESIAN_POINT ( 'NONE',  ( -9.311346830843410416, -51.41373841511900622, 1.033728595105000148 ) ) ;
#1109=CARTESIAN_POINT ( 'NONE',  ( -4.317466541193835106, -57.77653723152862142, 0.4415034884863752729 ) ) ;
#1113=CARTESIAN_POINT ( 'NONE',  ( -1.005393588828258133, -65.41824993351924888, -2.298700180912566449 ) ) ;
#1116=CARTESIAN_POINT ( 'NONE',  ( -6.227481695512121718, -59.47789623974718864, -0.5324849168858507564 ) ) ;
#1127=CARTESIAN_POINT ( 'NONE',  ( -8.362056880804429326, -51.09933645781752887, 2.533728595105000370 ) ) ;
#1128=CARTESIAN_POINT ( 'NONE',  ( -4.101849953070630050, -66.53066707031882743, 2.593177719986650143 ) ) ;
#1130=CIRCLE ( 'NONE', #3756, 0.5000000000000066613 ) ;
#1132=EDGE_CURVE ( 'NONE', #489, #4174, #1353, .T. ) ;
#1137=VECTOR ( 'NONE', #4984, 999.9999999999998863 ) ;
#1151=CARTESIAN_POINT ( 'NONE',  ( -1.432436674628349893, -67.38906872584260555, -2.752582849501530760 ) ) ;
#1158=CARTESIAN_POINT ( 'NONE',  ( 2.753836159791509974, -65.67748394244114252, 3.050484385245309849 ) ) ;
#1160=CARTESIAN_POINT ( 'NONE',  ( -4.053309352542619592, -65.19933310964161421, -0.8734501311131982471 ) ) ;
#1167=CARTESIAN_POINT ( 'NONE',  ( -1.985532163257450078, -53.63691243282757881, -1.870211432998861945 ) ) ;
#1169=CARTESIAN_POINT ( 'NONE',  ( 5.271413390890690387, -61.79997272665566044, -1.279516964844005900 ) ) ;
#1172=FILL_AREA_STYLE_COLOUR ( '', #4123 ) ;
#1173=FACE_OUTER_BOUND ( 'NONE', #4086, .T. ) ;
#1178=CARTESIAN_POINT ( 'NONE',  ( 10.30762257547189975, -51.58645851951763461, -2.495037190209991707 ) ) ;
#1180=EDGE_CURVE ( 'NONE', #1972, #123, #157, .T. ) ;
#1184=CARTESIAN_POINT ( 'NONE',  ( -5.205673437485017097, -63.09603712129732855, 1.507649522180431800 ) ) ;
#1185=CARTESIAN_POINT ( 'NONE',  ( 5.396949887678069935, -64.06165292293543700, 0.6913201402231599069 ) ) ;
#1187=EDGE_LOOP ( 'NONE', ( #5457, #3397, #3061, #6621, #1235 ) ) ;
#1188=CARTESIAN_POINT ( 'NONE',  ( -5.011296251047005157, -62.10358530323204462, 3.211213581958491492 ) ) ;
#1193=CARTESIAN_POINT ( 'NONE',  ( -5.689067437457130616, -61.48253059702771850, 3.675478928603590489 ) ) ;
#1194=DIRECTION ( 'NONE',  ( -0.2467992669038191478, 0.02032136184815930280, 0.9688535307818069153 ) ) ;
#1195=DIRECTION ( 'NONE',  ( 0.2223157560262044585, -0.6712493609847989262, 0.7071067811865449082 ) ) ;
#1202=CARTESIAN_POINT ( 'NONE',  ( -2.104778383727555102, -66.59261038346899397, 1.133408834283370137 ) ) ;
#1204=CARTESIAN_POINT ( 'NONE',  ( 2.734303695691099989, -65.14978033110251943, -1.014598242344157963 ) ) ;
#1205=B_SPLINE_CURVE_WITH_KNOTS ( 'NONE', 3,
 ( #5469, #3072, #7099, #5994, #5388, #2513, #4820, #4251, #4524, #1684 ),
 .UNSPECIFIED., .F., .F.,
 ( 4, 2, 2, 2, 4 ),
 ( 0.000000000000000000, 0.2500000000000002776, 0.5000000000000002220, 0.7500000000000001110, 1.000000000000000000 ),
 .UNSPECIFIED. ) ;
#1211=VECTOR ( 'NONE', #5626, 1000.000000000000114 ) ;
#1213=CARTESIAN_POINT ( 'NONE',  ( 3.403992074353090036, -54.97443010399496899, 2.224669212202579960 ) ) ;
#1219=CARTESIAN_POINT ( 'NONE',  ( 15.49911764349215026, -35.75048010860329839, 0.4975185951050001831 ) ) ;
#1220=CARTESIAN_POINT ( 'NONE',  ( 4.719984496330532409, -63.87667799492090381, 0.8260579302787993683 ) ) ;
#1221=CIRCLE ( 'NONE', #5427, 1.000000000000001110 ) ;
#1225=CARTESIAN_POINT ( 'NONE',  ( -5.078718092191791378, -62.12561931644285806, 3.276649263749329855 ) ) ;
#1227=CARTESIAN_POINT ( 'NONE',  ( -10.30756287540601868, -51.58645400917961865, 2.526284428608170263 ) ) ;
#1228=CARTESIAN_POINT ( 'NONE',  ( -1.799724466760814989, -66.07795133246216324, 3.315732812615050484 ) ) ;
#1229=CARTESIAN_POINT ( 'NONE',  ( -6.308476396955129850, -59.14191327212131455, -0.5142043607924547954 ) ) ;
#1235=ORIENTED_EDGE ( 'NONE', *, *, #2956, .F. ) ;
#1238=CIRCLE ( 'NONE', #2899, 1.000000000000001776 ) ;
#1239=AXIS2_PLACEMENT_3D ( 'NONE', #1108, #1751, #5323 ) ;
#1240=CARTESIAN_POINT ( 'NONE',  ( -3.381846796090564933, -54.21055914560344746, 0.1632119451740500493 ) ) ;
#1241=DIRECTION ( 'NONE',  ( 0.3144019573014849023, -0.9492899500389727629, 0.000000000000000000 ) ) ;
#1249=CARTESIAN_POINT ( 'NONE',  ( -14.81339646197689852, -34.80111785677370051, -0.4662714048949997969 ) ) ;
#1251=CARTESIAN_POINT ( 'NONE',  ( 6.643375263299909683, -62.64442119333418901, -2.502572238011808281 ) ) ;
#1254=CIRCLE ( 'NONE', #6772, 1.000000000000001110 ) ;
#1255=CARTESIAN_POINT ( 'NONE',  ( 1.080279179814437773, -65.65553934942860792, 2.784998920779040432 ) ) ;
#1258=DIRECTION ( 'NONE',  ( 2.290931512739800066E-16, 1.403768413105889815E-16, 1.000000000000000000 ) ) ;
#1260=EDGE_CURVE ( 'NONE', #327, #6872, #1366, .T. ) ;
#1262=DIRECTION ( 'NONE',  ( 0.000000000000000000, -0.7252565289002705917, -0.6884787340851793447 ) ) ;
#1263=AXIS2_PLACEMENT_3D ( 'NONE', #2069, #6089, #3989 ) ;
#1270=CARTESIAN_POINT ( 'NONE',  ( -2.889418079045375176, -55.97554976774797098, -0.4852521485111498389 ) ) ;
#1271=CARTESIAN_POINT ( 'NONE',  ( -6.239404450008960268, -62.05055862403510503, 1.429382062327010150 ) ) ;
#1282=CARTESIAN_POINT ( 'NONE',  ( -6.079305786110669629, -62.05959118544440400, 1.459294228111509995 ) ) ;
#1290=CARTESIAN_POINT ( 'NONE',  ( -4.721082446365287844, -64.53544812894149629, 1.276903664564835283 ) ) ;
#1291=CARTESIAN_POINT ( 'NONE',  ( -2.437747074861595031, -55.99259917890189797, 0.6173017669495700632 ) ) ;
#1294=CARTESIAN_POINT ( 'NONE',  ( -4.119466531011084065, -64.51282121827222227, -0.6949236412976698141 ) ) ;
#1296=CARTESIAN_POINT ( 'NONE',  ( -14.07431766324680034, -37.03265636863024923, 1.026284428608169819 ) ) ;
#1298=CARTESIAN_POINT ( 'NONE',  ( 3.069422284440780135, -65.49896014417400636, 0.9299900502622647780 ) ) ;
#1299=CARTESIAN_POINT ( 'NONE',  ( 5.929218414971320072, -62.35084102844776055, -1.530333388185332932 ) ) ;
#1301=ORIENTED_EDGE ( 'NONE', *, *, #4208, .F. ) ;
#1308=CARTESIAN_POINT ( 'NONE',  ( 1.600318488538475137, -66.74162401608067796, -1.164216807110747931 ) ) ;
#1322=CARTESIAN_POINT ( 'NONE',  ( -1.799724466760814989, -66.07795133246216324, 3.315732812615050484 ) ) ;
#1325=CARTESIAN_POINT ( 'NONE',  ( 5.537683946240698596, -62.28623092199279654, -1.376834937089043809 ) ) ;
#1326=CARTESIAN_POINT ( 'NONE',  ( 1.211170193666210038, -66.82801115824167937, 0.9562527914032201704 ) ) ;
#1327=CIRCLE ( 'NONE', #833, 0.9999999999999984457 ) ;
#1328=ORIENTED_EDGE ( 'NONE', *, *, #7328, .F. ) ;
#1331=DIRECTION ( 'NONE',  ( 0.3144066910790619951, 0.9492883822130741001, 0.000000000000000000 ) ) ;
#1333=CARTESIAN_POINT ( 'NONE',  ( 6.285636693253979779, -59.03245517747429716, 2.489777307435960374 ) ) ;
#1334=CARTESIAN_POINT ( 'NONE',  ( 4.697834216849050115, -63.19072998194386059, -1.190263883463073880 ) ) ;
#1335=CARTESIAN_POINT ( 'NONE',  ( -3.156642594714314853, -54.82761582543010093, 1.871643660998590697 ) ) ;
#1338=ORIENTED_EDGE ( 'NONE', *, *, #3346, .F. ) ;
#1342=CARTESIAN_POINT ( 'NONE',  ( 1.340549191775572080, -65.71857943717337491, -0.9252791854465649557 ) ) ;
#1344=ORIENTED_EDGE ( 'NONE', *, *, #6230, .F. ) ;
#1350=CARTESIAN_POINT ( 'NONE',  ( 6.285636693253979779, -59.03245517747429716, 2.489777307435960374 ) ) ;
#1353=CIRCLE ( 'NONE', #7115, 0.4999999999999985567 ) ;
#1357=CARTESIAN_POINT ( 'NONE',  ( 1.711268714270854918, -65.48362256684714566, -1.456162841279315945 ) ) ;
#1360=CIRCLE ( 'NONE', #865, 1.000000000000000444 ) ;
#1361=FACE_OUTER_BOUND ( 'NONE', #57, .T. ) ;
#1363=EDGE_CURVE ( 'NONE', #354, #2698, #1130, .T. ) ;
#1364=CARTESIAN_POINT ( 'NONE',  ( -1.736694270343700275, -54.87097428782529107, -2.111004410316564162 ) ) ;
#1366=CIRCLE ( 'NONE', #2320, 2.500000000000000444 ) ;
#1367=ORIENTED_EDGE ( 'NONE', *, *, #1439, .F. ) ;
#1368=DIRECTION ( 'NONE',  ( -0.3144019573014849023, 0.9492899500389726519, 0.000000000000000000 ) ) ;
#1371=CARTESIAN_POINT ( 'NONE',  ( -6.239404450008960268, -62.05055862403510503, 1.429382062327010150 ) ) ;
#1372=CIRCLE ( 'NONE', #2337, 0.9999999999999998890 ) ;
#1373=B_SPLINE_CURVE_WITH_KNOTS ( 'NONE', 3,
 ( #6229, #2296, #3314, #503 ),
 .UNSPECIFIED., .F., .F.,
 ( 4, 4 ),
 ( 0.000000000000000000, 1.000000000000000000 ),
 .UNSPECIFIED. ) ;
#1374=CIRCLE ( 'NONE', #2338, 0.9999999999999984457 ) ;
#1382=CARTESIAN_POINT ( 'NONE',  ( -2.585448123472324777, -55.65377943239024461, 0.04593497335228470535 ) ) ;
#1390=CARTESIAN_POINT ( 'NONE',  ( -5.799935258789999715, -64.30794688765904255, -0.8981536636440297094 ) ) ;
#1393=CARTESIAN_POINT ( 'NONE',  ( -3.268634523084565036, -65.37612200555487618, 3.404282007464019877 ) ) ;
#1396=CARTESIAN_POINT ( 'NONE',  ( -0.3939081796060026619, -54.66775925573097084, -2.032307766995797405 ) ) ;
#1399=CARTESIAN_POINT ( 'NONE',  ( 14.04314992439729970, -37.12718381969609993, 4.336808689942017736E-16 ) ) ;
#1403=CARTESIAN_POINT ( 'NONE',  ( -5.206993624623629913, -63.95781028998001716, 3.417603084305509853 ) ) ;
#1404=CARTESIAN_POINT ( 'NONE',  ( -1.735723365167664900, -67.19411771835910940, 0.9573769032209800134 ) ) ;
#1405=DIRECTION ( 'NONE',  ( 0.9492899500389726519, 0.3144019573014848468, 0.000000000000000000 ) ) ;
#1406=ORIENTED_EDGE ( 'NONE', *, *, #226, .T. ) ;
#1412=CARTESIAN_POINT ( 'NONE',  ( -1.334494426138621792, -66.80443255658586565, -3.107681693547102775 ) ) ;
#1413=CARTESIAN_POINT ( 'NONE',  ( -0.5105056437457926588, -54.21698483991842465, -0.08672375508415011702 ) ) ;
#1415=ORIENTED_EDGE ( 'NONE', *, *, #4679, .T. ) ;
#1421=CARTESIAN_POINT ( 'NONE',  ( -3.869447490927095057, -66.24422018797883993, 3.165055290057749993 ) ) ;
#1422=CARTESIAN_POINT ( 'NONE',  ( 14.97072768011073940, -34.32654753528365177, 2.597518595105000383 ) ) ;
#1423=CARTESIAN_POINT ( 'NONE',  ( -5.502354252718959948, -62.02724140920135198, 3.641858308670590016 ) ) ;
#1426=CARTESIAN_POINT ( 'NONE',  ( -5.784209743144936411, -61.27901533394182110, -2.583004453599333061 ) ) ;
#1429=DIRECTION ( 'NONE',  ( 0.3144019573014875113, -0.9492899500389717637, 0.000000000000000000 ) ) ;
#1431=CARTESIAN_POINT ( 'NONE',  ( 14.07443455944474131, -37.03272609524245240, -0.9950371902099899302 ) ) ;
#1432=DIRECTION ( 'NONE',  ( -0.2467992669038191478, 0.02032136184815930280, 0.9688535307818069153 ) ) ;
#1433=CARTESIAN_POINT ( 'NONE',  ( 2.986904076224405014, -66.15109244657664078, 2.931604786918900363 ) ) ;
#1435=CIRCLE ( 'NONE', #7326, 1.000000000000001776 ) ;
#1436=CARTESIAN_POINT ( 'NONE',  ( -7.069128816957480410, -61.66762450778810489, 2.866206824378770168 ) ) ;
#1439=EDGE_CURVE ( 'NONE', #1508, #3171, #23, .T. ) ;
#1444=CARTESIAN_POINT ( 'NONE',  ( 5.330483863435800274, -59.34891080545844488, 0.6651839376153853012 ) ) ;
#1446=ADVANCED_FACE ( 'NONE', ( #2279 ), #5096, .T. ) ;
#1447=CARTESIAN_POINT ( 'NONE',  ( -2.904120812423019782, -54.85523864424144591, 1.880038532258539563 ) ) ;
#1453=CARTESIAN_POINT ( 'NONE',  ( -14.97059744062764075, -34.32647288175419931, -2.566271404895000163 ) ) ;
#1455=CARTESIAN_POINT ( 'NONE',  ( -9.358272925367041140, -51.27205205187813419, 2.526284428608170263 ) ) ;
#1456=CARTESIAN_POINT ( 'NONE',  ( 2.080482015124565098, -66.54183146390657555, -1.221303033644861813 ) ) ;
#1462=CARTESIAN_POINT ( 'NONE',  ( -1.556563313654149905, -55.35434594439572464, -0.3959639196582302456 ) ) ;
#1466=CARTESIAN_POINT ( 'NONE',  ( -9.311346830843399758, -51.41373841511900622, 2.533728595105000370 ) ) ;
#1467=CARTESIAN_POINT ( 'NONE',  ( -6.575672653089386976, -62.62123098032723334, 2.148875912808684951 ) ) ;
#1473=ADVANCED_FACE ( 'NONE', ( #2323 ), #2360, .F. ) ;
#1476=CARTESIAN_POINT ( 'NONE',  ( -3.498019654714389581, -55.03494779767484602, -0.2490962732230048438 ) ) ;
#1479=CARTESIAN_POINT ( 'NONE',  ( -6.822623972396280934, -59.02239909983155286, -0.6330850349556997880 ) ) ;
#1480=CARTESIAN_POINT ( 'NONE',  ( 14.02750760687355935, -37.17441268192290238, 0.4975185951050001831 ) ) ;
#1483=ORIENTED_EDGE ( 'NONE', *, *, #1862, .F. ) ;
#1490=CARTESIAN_POINT ( 'NONE',  ( -5.091256589979570535, -61.80182140578926919, 1.697438579844070761 ) ) ;
#1492=CARTESIAN_POINT ( 'NONE',  ( 4.471690325102795072, -64.80734643215984647, 2.824010636486237846 ) ) ;
#1496=ORIENTED_EDGE ( 'NONE', *, *, #7023, .T. ) ;
#1505=CARTESIAN_POINT ( 'NONE',  ( 5.929218414971320072, -62.35084102844776055, -1.530333388185332932 ) ) ;
#1507=ORIENTED_EDGE ( 'NONE', *, *, #4985, .T. ) ;
#1508=VERTEX_POINT ( 'NONE', #6358 ) ;
#1510=CARTESIAN_POINT ( 'NONE',  ( -4.908132910216119527, -63.74296424117085991, -0.6604057789239049514 ) ) ;
#1519=CARTESIAN_POINT ( 'NONE',  ( 7.168555767344659380, -58.87994835687880624, 1.798531003845740051 ) ) ;
#1525=CARTESIAN_POINT ( 'NONE',  ( 2.576047814891095022, -64.81584722952422339, -0.4432308004904150223 ) ) ;
#1527=CARTESIAN_POINT ( 'NONE',  ( 5.863376863421286167, -57.99493907355560651, 0.3327841386862454565 ) ) ;
#1536=CARTESIAN_POINT ( 'NONE',  ( -6.722550792682009835, -58.60332661353002948, 1.487589938850535143 ) ) ;
#1538=EDGE_LOOP ( 'NONE', ( #6488, #977, #3851, #635, #4519, #6549 ) ) ;
#1544=DIRECTION ( 'NONE',  ( 0.2223191033124282123, 0.6712482523644723864, 0.7071067811865472397 ) ) ;
#1548=CARTESIAN_POINT ( 'NONE',  ( 15.49911764349215026, -35.75048010860329839, 0.4975185951050001831 ) ) ;
#1551=CARTESIAN_POINT ( 'NONE',  ( -6.634274853075190492, -62.58082626503517787, -0.8104611758546799161 ) ) ;
#1555=CARTESIAN_POINT ( 'NONE',  ( -14.49899450467539985, -35.75040780681265318, -0.4662714048949997969 ) ) ;
#1559=CARTESIAN_POINT ( 'NONE',  ( 5.193956696153660069, -59.28518064773341933, 2.254869812567109832 ) ) ;
#1561=CARTESIAN_POINT ( 'NONE',  ( -1.936202856841531039, -66.43606426736279502, -1.004513860088930732 ) ) ;
#1563=CARTESIAN_POINT ( 'NONE',  ( -6.217266535765080704, -62.33106447713396392, -2.754524245347104383 ) ) ;
#1570=FACE_OUTER_BOUND ( 'NONE', #2464, .T. ) ;
#1571=CARTESIAN_POINT ( 'NONE',  ( -14.63712380658832046, -36.05860345213164919, -4.315410310759999923 ) ) ;
#1573=CARTESIAN_POINT ( 'NONE',  ( 4.128395891713080523, -66.51223636356003510, -1.999098658498605019 ) ) ;
#1579=CARTESIAN_POINT ( 'NONE',  ( -5.714251477591489881, -57.46902543231049521, -0.4259505751857597389 ) ) ;
#1581=CYLINDRICAL_SURFACE ( 'NONE', #6976, 0.9999999999999984457 ) ;
#1586=AXIS2_PLACEMENT_3D ( 'NONE', #6147, #6449, #2490 ) ;
#1590=CARTESIAN_POINT ( 'NONE',  ( 14.63724902514210058, -34.60816281716094522, 2.969700630898919780 ) ) ;
#1591=DIRECTION ( 'NONE',  ( -0.08966155106958693943, -0.9959722919136836383, 0.000000000000000000 ) ) ;
#1592=CARTESIAN_POINT ( 'NONE',  ( 6.871427970997950219, -62.19563859352643931, -1.162241389626079702 ) ) ;
#1597=AXIS2_PLACEMENT_3D ( 'NONE', #3151, #1018, #7330 ) ;
#1599=CARTESIAN_POINT ( 'NONE',  ( -2.332017369136024865, -64.95045318432249815, -2.208845462231724177 ) ) ;
#1602=EDGE_CURVE ( 'NONE', #4768, #6909, #5340, .T. ) ;
#1605=CARTESIAN_POINT ( 'NONE',  ( -2.332017369136024865, -64.95045318432249815, -2.208845462231724177 ) ) ;
#1607=CARTESIAN_POINT ( 'NONE',  ( 5.091606878585934304, -64.16522473348585720, -1.423946029510006372 ) ) ;
#1613=CARTESIAN_POINT ( 'NONE',  ( -14.07431766324680034, -37.03265636863024923, 1.026284428608169819 ) ) ;
#1614=FACE_OUTER_BOUND ( 'NONE', #7315, .T. ) ;
#1615=CARTESIAN_POINT ( 'NONE',  ( -2.113079283527464991, -53.41662231759018198, -0.8523026345115048974 ) ) ;
#1616=AXIS2_PLACEMENT_3D ( 'NONE', #4322, #7215, #7098 ) ;
#1619=CARTESIAN_POINT ( 'NONE',  ( 6.162074140922939591, -62.32076522084695114, 2.666565443060120444 ) ) ;
#1624=ADVANCED_FACE ( 'NONE', ( #5905 ), #6534, .T. ) ;
#1628=CARTESIAN_POINT ( 'NONE',  ( 6.939112688521190009, -58.99009576954022549, 0.7806222117286002460 ) ) ;
#1634=CARTESIAN_POINT ( 'NONE',  ( -4.302337887170949671, -63.34626699285441020, 3.181678273100430054 ) ) ;
#1636=DIRECTION ( 'NONE',  ( 0.3144019573014853464, -0.9492899500389726519, -7.355227538141627568E-16 ) ) ;
#1637=CARTESIAN_POINT ( 'NONE',  ( -5.121204309455420045, -61.36711808260334067, 3.320501707867800523 ) ) ;
#1638=DIRECTION ( 'NONE',  ( 0.2223191033124283789, 0.6712482523644727195, 0.7071067811865466846 ) ) ;
#1639=CARTESIAN_POINT ( 'NONE',  ( -6.228944513034659458, -61.43090327710801546, -0.6374195285636679031 ) ) ;
#1640=CARTESIAN_POINT ( 'NONE',  ( 1.014503381694089823, -65.79094358639915185, 1.195300268011630029 ) ) ;
#1641=EDGE_CURVE ( 'NONE', #2620, #4300, #4234, .T. ) ;
#1644=EDGE_LOOP ( 'NONE', ( #1338, #7251, #6719, #4401, #501 ) ) ;
#1645=CARTESIAN_POINT ( 'NONE',  ( -14.63712380658832046, -35.33334692323139592, -3.626931576674818025 ) ) ;
#1648=CARTESIAN_POINT ( 'NONE',  ( 3.832282121198885338, -54.47902871778750722, 0.5155147207099053386 ) ) ;
#1658=CARTESIAN_POINT ( 'NONE',  ( 5.695730293278450596, -62.33055481056936742, -2.502481404895003259 ) ) ;
#1662=CARTESIAN_POINT ( 'NONE',  ( 1.773380156858839873, -67.30899524596459571, -0.8098396333890448551 ) ) ;
#1666=CARTESIAN_POINT ( 'NONE',  ( 4.837585924071849952, -61.97584320105620748, 1.412225657785534327 ) ) ;
#1671=CARTESIAN_POINT ( 'NONE',  ( 1.397902174090916105, -65.57924198930768966, 0.6644065888002452791 ) ) ;
#1673=CARTESIAN_POINT ( 'NONE',  ( -4.414126134886927844, -64.86522878795923930, -0.8472126198736709135 ) ) ;
#1675=VERTEX_POINT ( 'NONE', #4772 ) ;
#1684=CARTESIAN_POINT ( 'NONE',  ( 5.927764221498110331, -62.35749858221746678, -1.529935281190306862 ) ) ;
#1685=CARTESIAN_POINT ( 'NONE',  ( -6.519675230953620115, -62.56018929471859735, 1.797154853076760261 ) ) ;
#1687=AXIS2_PLACEMENT_3D ( 'NONE', #5281, #2936, #5206 ) ;
#1698=AXIS2_PLACEMENT_3D ( 'NONE', #3693, #3664, #6012 ) ;
#1699=ORIENTED_EDGE ( 'NONE', *, *, #3033, .F. ) ;
#1704=CARTESIAN_POINT ( 'NONE',  ( -1.855492712959899926, -67.28785520969887557, -0.6321745227666250022 ) ) ;
#1706=CARTESIAN_POINT ( 'NONE',  ( -5.107724228862107196, -62.13515610626047447, 3.301466892039410350 ) ) ;
#1711=CARTESIAN_POINT ( 'NONE',  ( -5.408997660349871062, -62.29959681528816873, 3.625047998704080232 ) ) ;
#1723=AXIS2_PLACEMENT_3D ( 'NONE', #2132, #6080, #2708 ) ;
#1726=DIRECTION ( 'NONE',  ( 0.000000000000000000, 0.000000000000000000, 1.000000000000000000 ) ) ;
#1728=CARTESIAN_POINT ( 'NONE',  ( -7.117253929586840222, -62.23044735776716152, 0.7381361199122749017 ) ) ;
#1748=CARTESIAN_POINT ( 'NONE',  ( 5.975049724055580214, -64.37929422792591083, -2.133092136665421190 ) ) ;
#1750=VERTEX_POINT ( 'NONE', #954 ) ;
#1751=DIRECTION ( 'NONE',  ( 0.9492899500389728740, 0.3144019573014844582, 0.000000000000000000 ) ) ;
#1755=CARTESIAN_POINT ( 'NONE',  ( 5.010558598472139913, -57.30068827582834956, 0.4001341763009204078 ) ) ;
#1757=DIRECTION ( 'NONE',  ( 0.000000000000000000, -0.7252570966694442678, 0.6884781359858920258 ) ) ;
#1758=VERTEX_POINT ( 'NONE', #834 ) ;
#1764=CARTESIAN_POINT ( 'NONE',  ( -3.760984799052800476, -54.43314106586858969, -1.957528877657078059 ) ) ;
#1765=LINE ( 'NONE', #1127, #5714 ) ;
#1766=CARTESIAN_POINT ( 'NONE',  ( -1.503553670228684913, -55.21328561235763743, -1.985649781529471802 ) ) ;
#1767=EDGE_CURVE ( 'NONE', #5892, #4812, #3131, .T. ) ;
#1781=CARTESIAN_POINT ( 'NONE',  ( -4.718809332073220730, -63.89081786388664597, 1.455152677735624289 ) ) ;
#1782=CARTESIAN_POINT ( 'NONE',  ( 3.942295684294244928, -66.34053734621645049, -3.017350621022677259 ) ) ;
#1784=ORIENTED_EDGE ( 'NONE', *, *, #2131, .T. ) ;
#1785=CARTESIAN_POINT ( 'NONE',  ( -4.949227490188758516, -62.08336044754862826, 3.140672163054920585 ) ) ;
#1789=CARTESIAN_POINT ( 'NONE',  ( 4.977719985769329725, -63.63849604921595216, 2.874328699340139792 ) ) ;
#1790=CARTESIAN_POINT ( 'NONE',  ( -1.592557218785495055, -66.68601476236933934, 1.076257986235874764 ) ) ;
#1791=DIRECTION ( 'NONE',  ( 0.9492899500389719858, 0.3144019573014870117, 0.000000000000000000 ) ) ;
#1793=EDGE_LOOP ( 'NONE', ( #2145, #2982, #3445, #1406, #538, #4127 ) ) ;
#1797=CARTESIAN_POINT ( 'NONE',  ( -5.707180516281660232, -57.33854382299282548, -2.489482313002657321 ) ) ;
#1806=CARTESIAN_POINT ( 'NONE',  ( -9.311346830843410416, -51.41373841511900622, 1.033728595105000148 ) ) ;
#1808=CARTESIAN_POINT ( 'NONE',  ( 14.63724902514210058, -36.05867701049984930, 4.346656902870709160 ) ) ;
#1811=CARTESIAN_POINT ( 'NONE',  ( -2.603817572988885054, -64.79915130424556935, -0.08835382460255962467 ) ) ;
#1813=CARTESIAN_POINT ( 'NONE',  ( 5.440311866380434402, -58.19481930409472881, 0.4849701219046175238 ) ) ;
#1815=FACE_OUTER_BOUND ( 'NONE', #1187, .T. ) ;
#1821=CARTESIAN_POINT ( 'NONE',  ( -2.909477865675369923, -55.29415281518058833, 1.990524098341705406 ) ) ;
#1822=CARTESIAN_POINT ( 'NONE',  ( -3.569041007005829602, -65.81017109676685095, 3.284668648760890264 ) ) ;
#1826=VERTEX_POINT ( 'NONE', #396 ) ;
#1829=AXIS2_PLACEMENT_3D ( 'NONE', #3249, #4316, #6605 ) ;
#1831=CARTESIAN_POINT ( 'NONE',  ( -1.432436674628349893, -67.38906872584260555, -2.752582849501530760 ) ) ;
#1842=CARTESIAN_POINT ( 'NONE',  ( 0.4291165664073187114, -54.21109657073610322, 2.063524181601441132 ) ) ;
#1843=AXIS2_PLACEMENT_3D ( 'NONE', #4436, #1726, #6839 ) ;
#1845=CARTESIAN_POINT ( 'NONE',  ( 2.818173014649640429, -55.92969527921476924, 1.989760685886134972 ) ) ;
#1848=DIRECTION ( 'NONE',  ( -0.3144066910790611624, -0.9492883822130743221, 0.000000000000000000 ) ) ;
#1849=CARTESIAN_POINT ( 'NONE',  ( 1.814912623942119829, -54.89591502488989505, 0.1965585422507683810 ) ) ;
#1850=CARTESIAN_POINT ( 'NONE',  ( -3.365275581743949918, -66.00192919971716776, -0.8990674732841750227 ) ) ;
#1856=CIRCLE ( 'NONE', #4149, 0.9999999999999998890 ) ;
#1859=CARTESIAN_POINT ( 'NONE',  ( 1.711268714270854918, -65.48362256684714566, -1.456162841279315945 ) ) ;
#1860=CARTESIAN_POINT ( 'NONE',  ( -1.974098099753330171, -66.57628266072889289, 3.196874607719439876 ) ) ;
#1862=EDGE_CURVE ( 'NONE', #1005, #5988, #1254, .T. ) ;
#1868=CARTESIAN_POINT ( 'NONE',  ( -6.776085205154060986, -62.52991726716069820, -2.400146893717961749 ) ) ;
#1872=ORIENTED_EDGE ( 'NONE', *, *, #1260, .T. ) ;
#1875=DIRECTION ( 'NONE',  ( -0.4328040977884316520, 0.5819352847797604200, 0.6884997728872834788 ) ) ;
#1876=CARTESIAN_POINT ( 'NONE',  ( -5.206993624623629913, -63.95781028998001716, 3.417603084305509853 ) ) ;
#1878=CARTESIAN_POINT ( 'NONE',  ( -5.710866809226770258, -58.90547762198222870, 1.725351541085619500 ) ) ;
#1879=CARTESIAN_POINT ( 'NONE',  ( -10.26063678088237907, -51.72814037242050489, 2.533728595105000370 ) ) ;
#1881=CARTESIAN_POINT ( 'NONE',  ( -1.847236269850647705, -65.97879705718997911, -0.8523026458531161031 ) ) ;
#1883=CARTESIAN_POINT ( 'NONE',  ( -14.97059744062764075, -34.32647288175419931, -2.566271404895000163 ) ) ;
#1887=CARTESIAN_POINT ( 'NONE',  ( 3.660823140336725068, -65.74644859602665292, -1.309095517728299907 ) ) ;
#1888=CARTESIAN_POINT ( 'NONE',  ( -4.574768583212910578, -63.39215034952142247, -2.605000795493774834 ) ) ;
#1890=DIRECTION ( 'NONE',  ( -0.08966155106958693943, -0.9959722919136836383, 0.000000000000000000 ) ) ;
#1896=CARTESIAN_POINT ( 'NONE',  ( 5.742131165818880056, -64.29439030986208081, -3.151051222873450630 ) ) ;
#1897=CARTESIAN_POINT ( 'NONE',  ( 5.927764221498110331, -62.35749858221746678, -1.529935281190306862 ) ) ;
#1900=EDGE_CURVE ( 'NONE', #4244, #6025, #7130, .T. ) ;
#1906=VERTEX_POINT ( 'NONE', #5673 ) ;
#1907=VECTOR ( 'NONE', #7151, 999.9999999999998863 ) ;
#1908=CARTESIAN_POINT ( 'NONE',  ( 5.113035703684060351, -58.96629286118465529, 0.1341944340671852032 ) ) ;
#1909=AXIS2_PLACEMENT_3D ( 'NONE', #6047, #2460, #315 ) ;
#1912=CARTESIAN_POINT ( 'NONE',  ( 0.01932788389254917402, -54.65463053036518914, 0.09165168851670162098 ) ) ;
#1915=FACE_OUTER_BOUND ( 'NONE', #5311, .T. ) ;
#1919=CARTESIAN_POINT ( 'NONE',  ( 3.403992074353090036, -54.97443010399496899, 2.224669212202579960 ) ) ;
#1926=CARTESIAN_POINT ( 'NONE',  ( -2.876828494605734754, -55.82398600891924190, -2.074803592940099861 ) ) ;
#1936=CARTESIAN_POINT ( 'NONE',  ( -2.148471732745839802, -67.07461398899560834, 3.078016402823839925 ) ) ;
#1938=TOROIDAL_SURFACE ( 'NONE', #4608, 1.500000000000000000, 1.000000000000000000 ) ;
#1941=CIRCLE ( 'NONE', #3870, 1.000000000000000444 ) ;
#1943=DIRECTION ( 'NONE',  ( 0.2223191033124283789, 0.6712482523644727195, 0.7071067811865466846 ) ) ;
#1945=CARTESIAN_POINT ( 'NONE',  ( 1.570963842414029976, -66.14661321919228953, 1.018783762524700265 ) ) ;
#1946=AXIS2_PLACEMENT_3D ( 'NONE', #4177, #5960, #780 ) ;
#1947=CYLINDRICAL_SURFACE ( 'NONE', #4726, 0.9999999999999991118 ) ;
#1949=CARTESIAN_POINT ( 'NONE',  ( 5.168836016896262819, -63.16969723543360260, -3.422093515887588477 ) ) ;
#1954=CIRCLE ( 'NONE', #3162, 1.000000000000000888 ) ;
#1956=TOROIDAL_SURFACE ( 'NONE', #2928, 1.500000000000000000, 1.000000000000000000 ) ;
#1959=CARTESIAN_POINT ( 'NONE',  ( -6.129265975028279634, -62.42766041111902098, -0.6909925287373350766 ) ) ;
#1961=CARTESIAN_POINT ( 'NONE',  ( -4.101849953070630050, -66.53066707031882743, 2.593177719986650143 ) ) ;
#1969=CARTESIAN_POINT ( 'NONE',  ( -2.527830428429834964, -65.26309079616396502, -2.780623214462280668 ) ) ;
#1970=CARTESIAN_POINT ( 'NONE',  ( 4.443182564071356033, -64.83719503748011448, 0.7261340252908324855 ) ) ;
#1971=ORIENTED_EDGE ( 'NONE', *, *, #4294, .T. ) ;
#1972=VERTEX_POINT ( 'NONE', #510 ) ;
#1978=DIRECTION ( 'NONE',  ( 0.1860016876085203719, -0.1636620475539280195, 0.9688230521603200529 ) ) ;
#1980=CARTESIAN_POINT ( 'NONE',  ( 6.802585521241110378, -58.92636561181245014, 2.370308086683080351 ) ) ;
#1985=CARTESIAN_POINT ( 'NONE',  ( 5.755397240816559901, -61.80640411027656000, 0.6650717595513898628 ) ) ;
#1989=DIRECTION ( 'NONE',  ( 0.9492899500389723189, 0.3144019573014865121, 0.000000000000000000 ) ) ;
#1990=CARTESIAN_POINT ( 'NONE',  ( -4.048469865975810933, -56.30416671985942401, -2.268338689207286318 ) ) ;
#1995=DIRECTION ( 'NONE',  ( -0.5224671166576538850, 0.8526594349512809368, 0.000000000000000000 ) ) ;
#1998=CARTESIAN_POINT ( 'NONE',  ( 2.080482015124565098, -66.54183146390657555, -1.221303033644861813 ) ) ;
#1999=CARTESIAN_POINT ( 'NONE',  ( -6.955550688080649913, -62.00810176775132021, 2.849210506046880642 ) ) ;
#2006=CARTESIAN_POINT ( 'NONE',  ( 1.276103242900551882, -55.15251840166065733, -1.809563881513800876 ) ) ;
#2008=CARTESIAN_POINT ( 'NONE',  ( -5.524031959655990143, -63.36203416574449676, 3.453224700803013025 ) ) ;
#2010=ORIENTED_EDGE ( 'NONE', *, *, #5795, .T. ) ;
#2012=CARTESIAN_POINT ( 'NONE',  ( 14.02750760687355935, -37.17441268192290238, 0.4975185951050001831 ) ) ;
#2015=CARTESIAN_POINT ( 'NONE',  ( 1.530679711083600125, -53.64394877353957014, -0.1027361406249600040 ) ) ;
#2019=CARTESIAN_POINT ( 'NONE',  ( 4.348279337280104961, -63.27746244242579365, -1.677170969482009832 ) ) ;
#2023=DIRECTION ( 'NONE',  ( 0.3128463504745289669, 0.9445772445362837777, 0.09950371902099817978 ) ) ;
#2032=CARTESIAN_POINT ( 'NONE',  ( -6.722550792682009835, -58.60332661353002948, 1.487589938850535143 ) ) ;
#2033=CARTESIAN_POINT ( 'NONE',  ( 9.327049558211379932, -51.36650955289220377, -1.499999999999997780 ) ) ;
#2035=EDGE_CURVE ( 'NONE', #4040, #7181, #1238, .T. ) ;
#2042=CARTESIAN_POINT ( 'NONE',  ( 5.178445921634760474, -62.11857673748845343, 0.8408583081513953950 ) ) ;
#2044=CARTESIAN_POINT ( 'NONE',  ( 3.702507633372579487, -65.47327791553946952, 0.7785861613390434588 ) ) ;
#2047=ORIENTED_EDGE ( 'NONE', *, *, #1363, .F. ) ;
#2052=CARTESIAN_POINT ( 'NONE',  ( -3.508682979600159957, -66.46637211483655960, 1.044995729122755179 ) ) ;
#2056=CLOSED_SHELL ( 'NONE', ( #3875, #1473, #2272, #2415, #5080, #1446, #2405, #3622, #6888, #4161, #3472, #5975, #5307, #5806, #5091, #374, #3746, #493, #1624, #3668, #4673, #879, #5647, #6337, #3440, #469, #5984, #2139, #903, #4392, #3140, #6553 ) ) ;
#2058=CARTESIAN_POINT ( 'NONE',  ( 3.331090576803830139, -65.95739139720836874, 0.8111086825117052035 ) ) ;
#2059=CIRCLE ( 'NONE', #520, 1.000000000000001110 ) ;
#2063=AXIS2_PLACEMENT_3D ( 'NONE', #4742, #103, #4639 ) ;
#2065=CIRCLE ( 'NONE', #2676, 2.499999999999997335 ) ;
#2069=CARTESIAN_POINT ( 'NONE',  ( -14.02739156872318027, -37.17434273187110705, -0.4662714048949997969 ) ) ;
#2072=UNCERTAINTY_MEASURE_WITH_UNIT (LENGTH_MEASURE( 1.000000000000000082E-05 ), #5276, 'distance_accuracy_value', 'NONE');
#2074=CARTESIAN_POINT ( 'NONE',  ( -14.97059744062764075, -34.32647288175419931, -2.566271404895000163 ) ) ;
#2076=CARTESIAN_POINT ( 'NONE',  ( -3.869447490927095057, -66.24422018797883993, 3.165055290057749993 ) ) ;
#2085=DIRECTION ( 'NONE',  ( 0.9492883822130744331, -0.3144066910790611624, 0.000000000000000000 ) ) ;
#2088=CARTESIAN_POINT ( 'NONE',  ( 4.115360779042029904, -63.19255852436059229, -2.695130055691413506 ) ) ;
#2090=CARTESIAN_POINT ( 'NONE',  ( 6.241005725948084226, -61.34940613753865080, 2.614218604193566886 ) ) ;
#2093=ORIENTED_EDGE ( 'NONE', *, *, #440, .T. ) ;
#2099=CARTESIAN_POINT ( 'NONE',  ( -5.640317424943829927, -64.23513207997909547, 3.298613272382739936 ) ) ;
#2102=CARTESIAN_POINT ( 'NONE',  ( 1.919155946380425082, -66.03927477571377835, -1.101811511879709826 ) ) ;
#2104=FACE_OUTER_BOUND ( 'NONE', #3497, .T. ) ;
#2109=CARTESIAN_POINT ( 'NONE',  ( -7.117253929586840222, -62.23044735776716152, 0.7381361199122749017 ) ) ;
#2111=ORIENTED_EDGE ( 'NONE', *, *, #4473, .F. ) ;
#2113=EDGE_CURVE ( 'NONE', #5269, #4768, #3138, .T. ) ;
#2116=CARTESIAN_POINT ( 'NONE',  ( -4.410792138572509735, -62.95272468751611683, 0.08690264739508006542 ) ) ;
#2118=CARTESIAN_POINT ( 'NONE',  ( 5.616564958267002083, -63.30981001137231345, -1.476279958498600609 ) ) ;
#2121=ORIENTED_EDGE ( 'NONE', *, *, #5795, .F. ) ;
#2126=CARTESIAN_POINT ( 'NONE',  ( 7.168555767344659380, -58.87994835687880624, 1.798531003845740051 ) ) ;
#2131=EDGE_CURVE ( 'NONE', #1089, #5892, #6051, .T. ) ;
#2132=CARTESIAN_POINT ( 'NONE',  ( -14.07431766324680034, -37.03265636863024923, 1.026284428608169819 ) ) ;
#2133=CARTESIAN_POINT ( 'NONE',  ( -1.892846266465454841, -54.28526762408564110, -0.1610563749503846620 ) ) ;
#2137=ORIENTED_EDGE ( 'NONE', *, *, #5252, .F. ) ;
#2138=ORIENTED_EDGE ( 'NONE', *, *, #1602, .F. ) ;
#2139=ADVANCED_FACE ( 'NONE', ( #6625 ), #3742, .T. ) ;
#2141=CARTESIAN_POINT ( 'NONE',  ( 14.49911764349215915, -35.75048010860329839, 2.597518595105000383 ) ) ;
#2142=CARTESIAN_POINT ( 'NONE',  ( -6.026503769217380402, -56.70691413961192495, -0.01483612153302480557 ) ) ;
#2145=ORIENTED_EDGE ( 'NONE', *, *, #1260, .F. ) ;
#2147=CARTESIAN_POINT ( 'NONE',  ( 1.475197934039484071, -55.33068667649028782, 1.900472455802885818 ) ) ;
#2152=CARTESIAN_POINT ( 'NONE',  ( -1.241878142352246028, -55.26848170174031338, 1.724521099399885182 ) ) ;
#2153=CARTESIAN_POINT ( 'NONE',  ( 14.63724902514211834, -35.33341991383040437, 3.658178766884810251 ) ) ;
#2156=CARTESIAN_POINT ( 'NONE',  ( -3.096824821213254975, -64.92072129780139278, 1.460348123614904514 ) ) ;
#2162=DIRECTION ( 'NONE',  ( 0.9492883822130744331, -0.3144066910790611624, 0.000000000000000000 ) ) ;
#2164=AXIS2_PLACEMENT_3D ( 'NONE', #6487, #2981, #1757 ) ;
#2166=CARTESIAN_POINT ( 'NONE',  ( -1.678659834933539985, -53.30027862203323252, 1.268182062803870247 ) ) ;
#2168=DIRECTION ( 'NONE',  ( 0.2223157560262044585, -0.6712493609847989262, 0.7071067811865449082 ) ) ;
#2170=CARTESIAN_POINT ( 'NONE',  ( 5.619938529503549773, -63.59344562873818774, 0.6343307546824898946 ) ) ;
#2175=ORIENTED_EDGE ( 'NONE', *, *, #6428, .F. ) ;
#2181=DIRECTION ( 'NONE',  ( -1.602374898470634869E-16, 1.442524254523139935E-17, 1.000000000000000000 ) ) ;
#2182=CARTESIAN_POINT ( 'NONE',  ( -3.760984799052800476, -54.43314106586858969, -1.957528877657078059 ) ) ;
#2185=CIRCLE ( 'NONE', #7358, 1.000000000000001776 ) ;
#2189=CARTESIAN_POINT ( 'NONE',  ( -4.871804169514039273, -62.10086352108921659, 3.270302337133240478 ) ) ;
#2195=CARTESIAN_POINT ( 'NONE',  ( 4.334569312604970470, -57.80406557947362245, -0.9730881136235148832 ) ) ;
#2197=DIRECTION ( 'NONE',  ( 0.3128416502900965290, -0.9445788350777319931, 0.09950339776592478924 ) ) ;
#2198=LINE ( 'NONE', #475, #7 ) ;
#2200=CARTESIAN_POINT ( 'NONE',  ( 3.594547628745600409, -65.86039197651267330, -3.372550074330296965 ) ) ;
#2201=ORIENTED_EDGE ( 'NONE', *, *, #1439, .T. ) ;
#2202=AXIS2_PLACEMENT_3D ( 'NONE', #5057, #1028, #5708 ) ;
#2210=CARTESIAN_POINT ( 'NONE',  ( -4.011890603535904987, -66.29221981733677183, 1.575336318554399595 ) ) ;
#2214=DIRECTION ( 'NONE',  ( 0.9492899500389723189, 0.3144019573014865121, 0.000000000000000000 ) ) ;
#2217=CARTESIAN_POINT ( 'NONE',  ( -5.895051854024569771, -62.45358532148892294, 3.505907163650189950 ) ) ;
#2229=CARTESIAN_POINT ( 'NONE',  ( -6.994430249510970476, -62.66069223349322925, -1.382237850844937777 ) ) ;
#2235=CARTESIAN_POINT ( 'NONE',  ( 4.334569312604970470, -57.80406557947362245, -0.9730881136235148832 ) ) ;
#2238=CARTESIAN_POINT ( 'NONE',  ( 4.469984187763964556, -63.33186444122004843, 2.519959534738519746 ) ) ;
#2250=CARTESIAN_POINT ( 'NONE',  ( 2.327488905229944560, -67.40324771348248589, -1.912586833593244773 ) ) ;
#2255=CARTESIAN_POINT ( 'NONE',  ( 13.49911764349216092, -35.75048010860329839, 0.4975185951050001831 ) ) ;
#2256=CARTESIAN_POINT ( 'NONE',  ( -15.49899450467540163, -35.75040780681265318, -2.566271404894997499 ) ) ;
#2259=ORIENTED_EDGE ( 'NONE', *, *, #3785, .T. ) ;
#2263=CARTESIAN_POINT ( 'NONE',  ( -1.564844514157090138, -53.52797147715784121, 0.2502733031487548443 ) ) ;
#2267=CARTESIAN_POINT ( 'NONE',  ( -4.747355111503322789, -62.01643032957871071, 2.629496613306467445 ) ) ;
#2269=DIRECTION ( 'NONE',  ( -0.2163384215910431896, -0.07165063022625259292, 0.9736857165079894072 ) ) ;
#2270=CARTESIAN_POINT ( 'NONE',  ( -4.423017985506799477, -63.40237279495851652, -1.015450938335749953 ) ) ;
#2272=ADVANCED_FACE ( 'NONE', ( #3351 ), #5663, .T. ) ;
#2273=CARTESIAN_POINT ( 'NONE',  ( 3.705224094368697152, -65.54171936622607575, -1.318943324162216824 ) ) ;
#2277=ORIENTED_EDGE ( 'NONE', *, *, #6598, .F. ) ;
#2279=FACE_OUTER_BOUND ( 'NONE', #158, .T. ) ;
#2282=CARTESIAN_POINT ( 'NONE',  ( -15.08175531864075047, -33.99084820126180517, -5.041145139047909396 ) ) ;
#2284=CARTESIAN_POINT ( 'NONE',  ( 1.647105754412080181, -53.29316706828264216, -0.6741030570719998005 ) ) ;
#2286=CIRCLE ( 'NONE', #243, 0.9999999999999998890 ) ;
#2287=ORIENTED_EDGE ( 'NONE', *, *, #4540, .T. ) ;
#2296=CARTESIAN_POINT ( 'NONE',  ( -5.071543166975963857, -62.10633079430171222, 1.661898009719716462 ) ) ;
#2297=CARTESIAN_POINT ( 'NONE',  ( 0.4505070138924615053, -66.21322040523499197, 1.114523354903560248 ) ) ;
#2298=CARTESIAN_POINT ( 'NONE',  ( -2.273841640848679901, -67.16083533941571204, 1.488471302465715018 ) ) ;
#2303=AXIS2_PLACEMENT_3D ( 'NONE', #1883, #6590, #1429 ) ;
#2306=DIRECTION ( 'NONE',  ( 0.3128463504745285229, 0.9445772445362839997, 0.09950371902099811039 ) ) ;
#2308=AXIS2_PLACEMENT_3D ( 'NONE', #193, #1258, #86 ) ;
#2309=CARTESIAN_POINT ( 'NONE',  ( 5.768687865266859838, -59.13854474313614418, 2.609246528188839509 ) ) ;
#2320=AXIS2_PLACEMENT_3D ( 'NONE', #1453, #4896, #4404 ) ;
#2322=EDGE_CURVE ( 'NONE', #4812, #489, #32, .T. ) ;
#2323=FACE_OUTER_BOUND ( 'NONE', #3428, .T. ) ;
#2325=CARTESIAN_POINT ( 'NONE',  ( 6.493768279116130415, -62.63809584774485018, -3.239169643854469705 ) ) ;
#2327=CARTESIAN_POINT ( 'NONE',  ( -1.435618805647706164, -65.69410370267330279, -0.7494494782121799981 ) ) ;
#2328=VERTEX_POINT ( 'NONE', #1879 ) ;
#2329=AXIS2_PLACEMENT_3D ( 'NONE', #6671, #314, #1432 ) ;
#2331=ORIENTED_EDGE ( 'NONE', *, *, #4170, .F. ) ;
#2334=EDGE_CURVE ( 'NONE', #6921, #210, #4235, .T. ) ;
#2335=DIRECTION ( 'NONE',  ( 0.000000000000000000, 0.000000000000000000, 1.000000000000000000 ) ) ;
#2337=AXIS2_PLACEMENT_3D ( 'NONE', #1431, #3616, #825 ) ;
#2338=AXIS2_PLACEMENT_3D ( 'NONE', #6911, #1943, #2902 ) ;
#2342=VERTEX_POINT ( 'NONE', #651 ) ;
#2348=CARTESIAN_POINT ( 'NONE',  ( 14.63724902514211834, -35.33341991383040437, 3.658178766884810251 ) ) ;
#2351=CARTESIAN_POINT ( 'NONE',  ( -4.748090069711009775, -62.01667038360579198, 2.533819555318849837 ) ) ;
#2354=CARTESIAN_POINT ( 'NONE',  ( 2.799893819535080208, -55.23287331081275653, 0.2233987335540700003 ) ) ;
#2355=CARTESIAN_POINT ( 'NONE',  ( -1.512046953658800152, -54.18079592905042574, 1.959428465566195543 ) ) ;
#2356=DIRECTION ( 'NONE',  ( 0.3128463504745289669, 0.9445772445362837777, 0.09950371902099887367 ) ) ;
#2360=PLANE ( 'NONE',  #7252 ) ;
#2362=CARTESIAN_POINT ( 'NONE',  ( -5.316774007586650086, -63.89131393482077925, 1.354123676545745170 ) ) ;
#2364=ORIENTED_EDGE ( 'NONE', *, *, #1900, .T. ) ;
#2365=EDGE_CURVE ( 'NONE', #5988, #4812, #2059, .T. ) ;
#2368=CARTESIAN_POINT ( 'NONE',  ( 14.49911764349215915, -35.75048010860329839, 0.4975185951050001831 ) ) ;
#2370=CARTESIAN_POINT ( 'NONE',  ( -4.748090069711009775, -62.01667038360579198, 2.533819555318849837 ) ) ;
#2371=CARTESIAN_POINT ( 'NONE',  ( -6.199032880790720235, -61.56120177486793210, 3.556545127952429830 ) ) ;
#2376=CARTESIAN_POINT ( 'NONE',  ( 1.576955190785845007, -65.26733347271304808, -2.474060432887700500 ) ) ;
#2380=ORIENTED_EDGE ( 'NONE', *, *, #7023, .F. ) ;
#2383=CARTESIAN_POINT ( 'NONE',  ( 4.841738599488129680, -63.57854475872899513, -1.322671891113719855 ) ) ;
#2384=CARTESIAN_POINT ( 'NONE',  ( -5.714251477591489881, -57.46902543231049521, -0.4259505751857597389 ) ) ;
#2385=DIRECTION ( 'NONE',  ( -0.4328040977884316520, 0.5819352847797604200, 0.6884997728872834788 ) ) ;
#2392=CARTESIAN_POINT ( 'NONE',  ( -5.951685856498870386, -64.29772444222471961, -2.487703520802049262 ) ) ;
#2396=AXIS2_PLACEMENT_3D ( 'NONE', #377, #1544, #2671 ) ;
#2402=FACE_OUTER_BOUND ( 'NONE', #5996, .T. ) ;
#2403=CARTESIAN_POINT ( 'NONE',  ( 5.360452058498115235, -63.64145676321751921, 2.745338867839514752 ) ) ;
#2405=ADVANCED_FACE ( 'NONE', ( #1570 ), #1947, .T. ) ;
#2406=EDGE_CURVE ( 'NONE', #2620, #6077, #986, .T. ) ;
#2408=CARTESIAN_POINT ( 'NONE',  ( 4.106052318423260239, -56.36209498175141874, 0.3538987277600479375 ) ) ;
#2411=CARTESIAN_POINT ( 'NONE',  ( -6.176129832103540274, -61.75772637036916279, 1.476179264717100370 ) ) ;
#2413=CARTESIAN_POINT ( 'NONE',  ( -4.759129193302329419, -62.02058092981934578, 2.720659859784867241 ) ) ;
#2415=ADVANCED_FACE ( 'NONE', ( #4297 ), #1938, .T. ) ;
#2418=CARTESIAN_POINT ( 'NONE',  ( -5.794328821513979655, -59.26142744441108334, -0.3953236866292048068 ) ) ;
#2419=CARTESIAN_POINT ( 'NONE',  ( 5.416018991692120643, -63.93240027730202968, 2.754852738177090643 ) ) ;
#2420=CARTESIAN_POINT ( 'NONE',  ( -14.49899450467539985, -35.75040780681265318, -2.566271404894997499 ) ) ;
#2423=EDGE_LOOP ( 'NONE', ( #3444, #4285, #6104, #5051, #2331 ) ) ;
#2425=DIRECTION ( 'NONE',  ( 0.3128416502900965290, -0.9445788350777318820, 0.09950339776592408148 ) ) ;
#2429=CARTESIAN_POINT ( 'NONE',  ( 1.647567807763375081, -53.54661630431167652, -1.692287459705078101 ) ) ;
#2446=CARTESIAN_POINT ( 'NONE',  ( -2.889418079045375176, -55.97554976774797098, -0.4852521485111498389 ) ) ;
#2450=CARTESIAN_POINT ( 'NONE',  ( 5.071800925510882685, -62.16193033951381608, -3.298373296383677822 ) ) ;
#2451=CARTESIAN_POINT ( 'NONE',  ( -5.712169679815763068, -59.50909061234685993, -0.3802802853964926122 ) ) ;
#2452=CIRCLE ( 'NONE', #2699, 1.000000000000000444 ) ;
#2460=DIRECTION ( 'NONE',  ( 0.2223157560262044585, -0.6712493609847989262, 0.7071067811865449082 ) ) ;
#2461=CARTESIAN_POINT ( 'NONE',  ( 4.980378365057210210, -62.14367890036703557, -3.355420260138584521 ) ) ;
#2462=CARTESIAN_POINT ( 'NONE',  ( -6.599700898649300207, -61.96243991103532522, 3.420662994399620072 ) ) ;
#2464=EDGE_LOOP ( 'NONE', ( #5179, #6528, #4468, #3270, #3678, #6357 ) ) ;
#2472=CARTESIAN_POINT ( 'NONE',  ( -5.509265921604280081, -56.99747518668161206, -0.3692125993829896702 ) ) ;
#2475=EDGE_CURVE ( 'NONE', #6355, #327, #146, .T. ) ;
#2484=CARTESIAN_POINT ( 'NONE',  ( -5.155987128177820900, -61.76400128369626685, 1.194474120832875519 ) ) ;
#2487=CARTESIAN_POINT ( 'NONE',  ( -1.869726328446417840, -65.97170341743343158, -2.950226656714010964 ) ) ;
#2488=CARTESIAN_POINT ( 'NONE',  ( 5.608858804484560423, -63.72364544018660126, -1.429200976399037870 ) ) ;
#2490=DIRECTION ( 'NONE',  ( 0.1860016876085203441, -0.1636620475539279917, 0.9688230521603200529 ) ) ;
#2494=CARTESIAN_POINT ( 'NONE',  ( -5.563801105733269914, -63.69014839564722763, 1.341242183458755344 ) ) ;
#2495=CARTESIAN_POINT ( 'NONE',  ( 4.396896920912054973, -63.41639021975223045, -3.266830536337445245 ) ) ;
#2496=CARTESIAN_POINT ( 'NONE',  ( 5.661113010068490325, -57.37064013373739613, 2.401523511004880262 ) ) ;
#2505=CARTESIAN_POINT ( 'NONE',  ( -1.503553670228684913, -55.21328561235763743, -1.985649781529471802 ) ) ;
#2512=CARTESIAN_POINT ( 'NONE',  ( 14.07443455944474131, -37.03272609524245240, -0.9950371902099899302 ) ) ;
#2513=CARTESIAN_POINT ( 'NONE',  ( 5.228045628684117041, -62.14238301185224600, -1.625324146853510232 ) ) ;
#2514=CARTESIAN_POINT ( 'NONE',  ( 6.075450823322679383, -63.85990335785957228, 0.5148622082158803570 ) ) ;
#2519=CARTESIAN_POINT ( 'NONE',  ( -5.101403815575769940, -63.43555091703197490, 1.460123530859765317 ) ) ;
#2523=CARTESIAN_POINT ( 'NONE',  ( 2.167449936104646646, -65.91963042757416247, -3.186153502388756831 ) ) ;
#2530=CARTESIAN_POINT ( 'NONE',  ( 1.402950248545461909, -54.15620739517822813, 0.01614447287717020105 ) ) ;
#2531=CARTESIAN_POINT ( 'NONE',  ( -5.971666637568279867, -56.84728173661435591, 1.574849794282134896 ) ) ;
#2534=ORIENTED_EDGE ( 'NONE', *, *, #2721, .F. ) ;
#2535=AXIS2_PLACEMENT_3D ( 'NONE', #1480, #4950, #3771 ) ;
#2537=DIRECTION ( 'NONE',  ( 0.3128463504745289669, 0.9445772445362837777, 0.09950371902099887367 ) ) ;
#2539=CARTESIAN_POINT ( 'NONE',  ( -5.010373352768399791, -62.05347898811812968, 1.680690861613699516 ) ) ;
#2540=CARTESIAN_POINT ( 'NONE',  ( 0.5703416102740482829, -66.66371095433655114, 3.059999667144134960 ) ) ;
#2544=APPLICATION_CONTEXT ( 'automotive_design' ) ;
#2549=DIRECTION ( 'NONE',  ( 0.3128416502900970286, -0.9445788350777319931, 0.09950339776592319330 ) ) ;
#2551=CARTESIAN_POINT ( 'NONE',  ( -1.892846266465454841, -54.28526762408564110, -0.1610563749503846620 ) ) ;
#2554=B_SPLINE_CURVE_WITH_KNOTS ( 'NONE', 3,
 ( #2351, #2267, #2413, #6862, #547, #2831, #1785, #1188, #6943, #2977, #1225, #3508, #3470, #1706, #5828, #658, #2945, #124, #5260 ),
 .UNSPECIFIED., .F., .F.,
 ( 4, 2, 2, 2, 2, 1, 2, 2, 2, 4 ),
 ( 0.000000000000000000, 0.1250000000000031641, 0.2500000000000063283, 0.3750000000000094924, 0.4375000000000104916, 0.4687500000000099920, 0.4843750000000104361, 0.5000000000000108802, 0.7500000000000054401, 1.000000000000000000 ),
 .UNSPECIFIED. ) ;
#2559=CARTESIAN_POINT ( 'NONE',  ( 5.661089107917369745, -62.15448909529578003, 2.785446686898291002 ) ) ;
#2560=AXIS2_PLACEMENT_3D ( 'NONE', #3482, #5074, #4022 ) ;
#2563=CARTESIAN_POINT ( 'NONE',  ( -3.419625075451274920, -55.70566946813526954, -0.1180528406916061396 ) ) ;
#2567=CIRCLE ( 'NONE', #3884, 1.000000000000000000 ) ;
#2573=CARTESIAN_POINT ( 'NONE',  ( 3.059030343303239974, -54.77303090793805040, 0.1039292770420399137 ) ) ;
#2575=CARTESIAN_POINT ( 'NONE',  ( -3.132958547045754827, -66.67000521241658362, -1.075502346145061683 ) ) ;
#2578=ORIENTED_EDGE ( 'NONE', *, *, #6874, .F. ) ;
#2580=CARTESIAN_POINT ( 'NONE',  ( -15.49899450467540163, -35.75040780681265318, -2.566271404894997499 ) ) ;
#2582=CARTESIAN_POINT ( 'NONE',  ( -4.132930949989339631, -63.16624423302310021, 2.163545901557570428 ) ) ;
#2584=CARTESIAN_POINT ( 'NONE',  ( 5.080240932704482404, -56.71201383481658809, 0.2543090620532720836 ) ) ;
#2586=ORIENTED_EDGE ( 'NONE', *, *, #4208, .T. ) ;
#2587=ORIENTED_EDGE ( 'NONE', *, *, #5324, .F. ) ;
#2592=CARTESIAN_POINT ( 'NONE',  ( -3.773574383489684880, -54.58470482469731877, -0.3679774332281250393 ) ) ;
#2593=DIRECTION ( 'NONE',  ( 0.3144019573014853464, -0.9492899500389726519, -7.355227538141627568E-16 ) ) ;
#2594=CARTESIAN_POINT ( 'NONE',  ( -4.596296085628660322, -63.12536419624139938, 1.105086706205665070 ) ) ;
#2599=CARTESIAN_POINT ( 'NONE',  ( 1.408436980921016657, -54.83301260727528614, -1.927461220960678512 ) ) ;
#2602=CARTESIAN_POINT ( 'NONE',  ( 9.311407240687648468, -51.41373841511900622, -2.502481404895003259 ) ) ;
#2603=DIRECTION ( 'NONE',  ( 0.3128416502900974727, -0.9445788350777317710, 0.09950339776592416474 ) ) ;
#2606=CARTESIAN_POINT ( 'NONE',  ( 1.316624512147740012, -66.75104842734066324, 3.019790780136459851 ) ) ;
#2608=CARTESIAN_POINT ( 'NONE',  ( -2.296719424894785089, -67.41321183710302023, 2.506665444375390184 ) ) ;
#2615=CARTESIAN_POINT ( 'NONE',  ( -1.180326523133921945, -55.13093161118004559, 0.1348352173942452270 ) ) ;
#2617=CARTESIAN_POINT ( 'NONE',  ( 2.938012310013605966, -66.01711806483515943, 2.928912350400478370 ) ) ;
#2618=VERTEX_POINT ( 'NONE', #6326 ) ;
#2620=VERTEX_POINT ( 'NONE', #523 ) ;
#2625=CARTESIAN_POINT ( 'NONE',  ( -1.318626809553760104, -67.28799943462540512, -1.163043645407473958 ) ) ;
#2630=CARTESIAN_POINT ( 'NONE',  ( -3.156642594714314853, -54.82761582543010093, 1.871643660998590697 ) ) ;
#2642=CARTESIAN_POINT ( 'NONE',  ( 3.318166867071405068, -54.31318850506334428, -0.01554017946999016950 ) ) ;
#2650=CARTESIAN_POINT ( 'NONE',  ( 2.959376181595404720, -55.87711464508088710, 0.4000749283577051951 ) ) ;
#2652=CARTESIAN_POINT ( 'NONE',  ( 5.623883274648896702, -63.28098278875869909, 0.6212483640015137309 ) ) ;
#2655=CARTESIAN_POINT ( 'NONE',  ( -5.707180516281660232, -57.33854382299282548, -2.489482313002657321 ) ) ;
#2661=CIRCLE ( 'NONE', #1239, 2.500000000000000000 ) ;
#2662=CARTESIAN_POINT ( 'NONE',  ( -14.07431766324680034, -37.03265636863024923, 1.026284428608169819 ) ) ;
#2664=CARTESIAN_POINT ( 'NONE',  ( 5.676184037656430093, -63.13711808556965366, -1.485967351095627720 ) ) ;
#2665=VERTEX_POINT ( 'NONE', #6924 ) ;
#2666=AXIS2_PLACEMENT_3D ( 'NONE', #1296, #3084, #6479 ) ;
#2671=DIRECTION ( 'NONE',  ( 0.9492883822130743221, -0.3144066910790611069, 0.000000000000000000 ) ) ;
#2675=ORIENTED_EDGE ( 'NONE', *, *, #943, .F. ) ;
#2676=AXIS2_PLACEMENT_3D ( 'NONE', #4426, #2085, #995 ) ;
#2682=CARTESIAN_POINT ( 'NONE',  ( 3.691078954254495059, -54.53160935192415337, 2.105200478230089267 ) ) ;
#2690=AXIS2_PLACEMENT_3D ( 'NONE', #5976, #4797, #1331 ) ;
#2693=CARTESIAN_POINT ( 'NONE',  ( 2.837825173909910514, -64.65273986048342181, -2.563810374748431098 ) ) ;
#2698=VERTEX_POINT ( 'NONE', #214 ) ;
#2699=AXIS2_PLACEMENT_3D ( 'NONE', #2602, #4912, #6451 ) ;
#2706=CARTESIAN_POINT ( 'NONE',  ( -6.728394430327000464, -62.68905628767773663, 2.815217869383099814 ) ) ;
#2708=DIRECTION ( 'NONE',  ( -0.2467992669038191755, 0.02032136184815236737, 0.9688535307818070264 ) ) ;
#2709=CARTESIAN_POINT ( 'NONE',  ( -2.642495264810874822, -65.73545435749777255, -0.8365618114303696728 ) ) ;
#2712=CARTESIAN_POINT ( 'NONE',  ( -6.020862807469525180, -62.43680103905647627, 1.595792085579407216 ) ) ;
#2716=CARTESIAN_POINT ( 'NONE',  ( -6.177019684192219806, -63.92521542081036756, -0.3671906505365997164 ) ) ;
#2719=DIRECTION ( 'NONE',  ( 2.290931512739800066E-16, 1.403768413105889815E-16, 1.000000000000000000 ) ) ;
#2720=CARTESIAN_POINT ( 'NONE',  ( -1.308638315835680022, -65.34704488060808103, -0.1780822347184347620 ) ) ;
#2721=EDGE_CURVE ( 'NONE', #4944, #7318, #3400, .T. ) ;
#2724=CARTESIAN_POINT ( 'NONE',  ( 4.676675357529780364, -57.90541686953501710, 2.165367849443769810 ) ) ;
#2727=ORIENTED_EDGE ( 'NONE', *, *, #3679, .F. ) ;
#2732=ORIENTED_EDGE ( 'NONE', *, *, #707, .F. ) ;
#2734=CARTESIAN_POINT ( 'NONE',  ( 6.939112688521190009, -58.99009576954022549, 0.7806222117286002460 ) ) ;
#2738=CARTESIAN_POINT ( 'NONE',  ( 1.785462125252589960, -54.25404267560509908, 2.136629312307830375 ) ) ;
#2743=DIRECTION ( 'NONE',  ( -1.602374898470634869E-16, 1.442524254523139935E-17, 1.000000000000000000 ) ) ;
#2744=CARTESIAN_POINT ( 'NONE',  ( 6.134453413605339911, -63.99854120705014537, -1.074823505768055742 ) ) ;
#2745=CARTESIAN_POINT ( 'NONE',  ( 15.08188723176695056, -33.26566631243199623, 4.383914193272020476 ) ) ;
#2749=CARTESIAN_POINT ( 'NONE',  ( -5.038070929474960380, -61.61169989543196834, 3.303768584289609844 ) ) ;
#2753=CARTESIAN_POINT ( 'NONE',  ( -1.429016193381374089, -55.57463605963037168, -1.413872718151093721 ) ) ;
#2756=ORIENTED_EDGE ( 'NONE', *, *, #226, .F. ) ;
#2759=ORIENTED_EDGE ( 'NONE', *, *, #4905, .F. ) ;
#2766=CARTESIAN_POINT ( 'NONE',  ( -6.487383171013251015, -57.01613561570176358, -1.117195879216653864 ) ) ;
#2767=ORIENTED_EDGE ( 'NONE', *, *, #4549, .T. ) ;
#2771=( NAMED_UNIT ( * ) PLANE_ANGLE_UNIT ( ) SI_UNIT ( $, .RADIAN. ) );
#2772=CARTESIAN_POINT ( 'NONE',  ( 3.059030343303239974, -54.77303090793805040, 0.1039292770420399137 ) ) ;
#2775=CARTESIAN_POINT ( 'NONE',  ( 14.63724902514210058, -35.33341991383040437, 3.658178766884820465 ) ) ;
#2784=CARTESIAN_POINT ( 'NONE',  ( 3.832282121198885338, -54.47902871778750722, 0.5155147207099053386 ) ) ;
#2791=CARTESIAN_POINT ( 'NONE',  ( 2.837825173909910514, -64.65273986048342181, -2.563810374748431098 ) ) ;
#2796=CARTESIAN_POINT ( 'NONE',  ( -2.678905510920184696, -65.04233304593640241, 0.9295552878624004922 ) ) ;
#2799=ORIENTED_EDGE ( 'NONE', *, *, #162, .F. ) ;
#2808=CARTESIAN_POINT ( 'NONE',  ( 13.12514617723165955, -36.71831940416339535, -0.9950371902099899302 ) ) ;
#2810=CARTESIAN_POINT ( 'NONE',  ( -2.296719424894785089, -67.41321183710302023, 2.506665444375390184 ) ) ;
#2812=ORIENTED_EDGE ( 'NONE', *, *, #4038, .T. ) ;
#2815=( LENGTH_UNIT ( ) NAMED_UNIT ( * ) SI_UNIT ( .MILLI., .METRE. ) );
#2817=CIRCLE ( 'NONE', #5119, 0.9999999999999998890 ) ;
#2820=CARTESIAN_POINT ( 'NONE',  ( 13.49911764349216092, -35.75048010860329839, 2.597518595105000383 ) ) ;
#2828=CARTESIAN_POINT ( 'NONE',  ( -6.840816475388580287, -61.57127885238590892, 1.848044054229609934 ) ) ;
#2831=CARTESIAN_POINT ( 'NONE',  ( -4.908491537261493676, -62.07009784221990856, 3.085829421542757522 ) ) ;
#2832=CARTESIAN_POINT ( 'NONE',  ( 9.358334193258830425, -51.27205182843857045, -2.495037190209989930 ) ) ;
#2834=CARTESIAN_POINT ( 'NONE',  ( -4.871804169514039273, -62.10086352108921659, 3.270302337133240478 ) ) ;
#2836=CARTESIAN_POINT ( 'NONE',  ( -5.046087304442132826, -64.12077430324966087, -0.7947617384407686947 ) ) ;
#2839=ORIENTED_EDGE ( 'NONE', *, *, #3335, .F. ) ;
#2842=ORIENTED_EDGE ( 'NONE', *, *, #7245, .T. ) ;
#2846=CARTESIAN_POINT ( 'NONE',  ( -6.955550688080649913, -62.00810176775132021, 2.849210506046880642 ) ) ;
#2860=CARTESIAN_POINT ( 'NONE',  ( -3.723298236168965047, -66.76642012610518861, 0.4732191326009700938 ) ) ;
#2865=CARTESIAN_POINT ( 'NONE',  ( -9.311346830843410416, -51.41373841511902043, 1.533728595105000370 ) ) ;
#2868=CARTESIAN_POINT ( 'NONE',  ( 4.897692307440769888, -62.02301377339387756, -1.765793165935516829 ) ) ;
#2869=CIRCLE ( 'NONE', #7079, 1.000000000000001776 ) ;
#2873=EDGE_CURVE ( 'NONE', #1758, #4244, #2065, .T. ) ;
#2879=CARTESIAN_POINT ( 'NONE',  ( 5.608858804484560423, -63.72364544018660126, -1.429200976399037870 ) ) ;
#2881=CARTESIAN_POINT ( 'NONE',  ( -5.294444503516980483, -61.70453834742492916, -0.3952116983248150084 ) ) ;
#2883=ORIENTED_EDGE ( 'NONE', *, *, #4540, .F. ) ;
#2886=B_SPLINE_SURFACE_WITH_KNOTS ( 'NONE', 3, 3, ( 
 ( #7084, #3015, #3551, #5373, #6979, #5229, #1822, #1860, #691, #4694, #2419, #5899, #2949, #2496, #1919, #3620, #2355, #1335, #3515, #4227, #1271, #6948, #6526, #1790, #2980, #5331, #4121, #5867, #5837, #170, #4083, #6425, #95, #6385, #2384, #1229, #768, #5294, #663, #5264, #128, #4729, #3059, #6454, #1299 ),
 ( #724, #2462, #205, #388, #6676, #6159, #2076, #6564, #6049, #3770, #4274, #916, #5525, #873, #2682, #6595, #278, #5441, #2531, #2032, #6010, #3088, #829, #1404, #3692, #350, #317, #6093, #6709, #4343, #2642, #4916, #3124, #6631, #4388, #1479, #1551, #4949, #2575, #7160, #7270, #5402, #3204, #4881, #4836 ),
 ( #1436, #1999, #4307, #3727, #239, #7124, #1961, #2608, #3168, #5494, #7197, #7232, #1519, #3805, #3841, #6126, #949, #3241, #5558, #4989, #2109, #4421, #2860, #432, #4502, #3957, #3882, #1066, #8, #5060, #544, #6268, #6743, #5021, #6198, #6232, #2229, #5143, #7305, #505, #6784, #1030, #1748, #3354, #6311 ),
 ( #2828, #7420, #4613, #5667, #1105, #5632, #5175, #2298, #984, #3317, #7386, #465, #1628, #4000, #2784, #3279, #2263, #4572, #2142, #4044, #5103, #2716, #6906, #1704, #1662, #4536, #2744, #1592, #6859, #5598, #4456, #7342, #575, #2182, #3920, #5746, #6820, #3393, #5710, #1151, #3434, #1782, #2942, #685, #6477 ),
 ( #4792, #2411, #7045, #3503, #5319, #713, #4109, #154, #1326, #3007, #1185, #754, #6415, #5823, #4718, #654, #5928, #4154, #7006, #3049, #5257, #7076, #1850, #6447, #5364, #197, #2488, #6345, #3467, #5780, #608, #2896, #54, #476, #2655, #1077, #1563, #6103, #3933, #5534, #3852, #2200, #6171, #1001, #4960 ),
 ( #3292, #6687, #517, #5610, #362, #4515, #2156, #6797, #1640, #7397, #4356, #6999, #593, #4061, #632, #31, #2922, #4191, #6484, #204, #2881, #5372, #6362, #2327, #5197, #1204, #1334, #1169, #5241, #6927, #7053, #3058, #1766, #5765, #3619, #3486, #5938, #1888, #766, #5805, #4640, #73, #2495, #3453, #2461 ),
 ( #4762, #3321, #509, #7002, #4508, #85, #5817, #6204, #4461, #5636, #5671, #1666, #4683, #6747, #7390, #6236, #470, #1291, #1109, #6824, #5064, #1035, #1811, #2720, #3573, #3498, #4715, #3924, #3962, #2235, #648, #5285, #4106, #436, #6964, #3889, #3360, #2938, #1599, #5253, #2376, #2791, #116, #1070, #7346 ),
 ( #6273, #2749, #5026, #2189, #6790, #1634, #6409, #5109, #1255, #7309, #5857, #681, #4542, #2971, #1845, #2147, #4258, #4329, #5429, #5922, #2484, #2594, #708, #6000, #3043, #5313, #4183, #855, #1908, #4788, #6474, #7072, #1462, #2446, #5887, #3078, #3649, #4752, #192, #817, #1357, #4218, #2019, #7149, #262 ),
 ( #2999, #6620, #1423, #306, #149, #6510, #1393, #1322, #5968, #4902, #788, #2559, #3681, #3607, #7040, #747, #5391, #7106, #4867, #1878, #228, #2519, #5360, #4825, #1945, #3714, #7185, #1985, #4296, #6584, #6552, #3111, #6038, #3153, #5479, #5655, #3755, #1510, #2709, #940, #2102, #6771, #6149, #6082, #5047 ),
 ( #6810, #3827, #3191, #2217, #4484, #495, #905, #3795, #5013, #3227, #4411, #1619, #973, #5515, #7331, #2738, #338, #2630, #3263, #4939, #4527, #3909, #4445, #7296, #5547, #2058, #2170, #7224, #7372, #6730, #2772, #7262, #2133, #5584, #1579, #1057, #6223, #4373, #3345, #6664, #6702, #3866, #6117, #6185, #1019 ) ),
 .UNSPECIFIED., .T., .F., .F.,
 ( 4, 2, 2, 2, 4 ),
 ( 4, 3, 2, 2, 2, 2, 2, 2, 2, 2, 2, 2, 2, 2, 2, 2, 2, 2, 2, 2, 2, 4 ),
 ( 0.000000000000000000, 0.2500000000000000000, 0.5000000000000000000, 0.7500000000000000000, 1.000000000000000000 ),
 ( -0.01000000000000000021, 0.000000000000000000, 0.02628634692406570106, 0.07896140836526269191, 0.1315838524972270107, 0.1842089079736879964, 0.2368304666025229932, 0.2894621644501310098, 0.3421084969797454911, 0.3947501728568885149, 0.4473769119526340154, 0.5000000000000000000, 0.5526230880473660401, 0.6052498271431119292, 0.6578915030202550085, 0.7105378355498690457, 0.7631695333974770623, 0.8157910920263119481, 0.8684161475027730726, 0.9210385916347370028, 0.9737136530759340491, 1.000000000000000000 ),
 .UNSPECIFIED. ) ;
#2895=LINE ( 'NONE', #1104, #4577 ) ;
#2896=CARTESIAN_POINT ( 'NONE',  ( 1.531562167974070077, -54.12800115838471271, -2.047325108518057935 ) ) ;
#2899=AXIS2_PLACEMENT_3D ( 'NONE', #4509, #4543, #3438 ) ;
#2901=TOROIDAL_SURFACE ( 'NONE', #3023, 1.500000000000000000, 1.000000000000000000 ) ;
#2902=DIRECTION ( 'NONE',  ( 0.000000000000000000, -0.7252570966694443788, 0.6884781359858918037 ) ) ;
#2907=CARTESIAN_POINT ( 'NONE',  ( -5.502354252718959948, -62.02724140920135198, 3.641858308670590016 ) ) ;
#2915=DIRECTION ( 'NONE',  ( -0.9492899500389724299, -0.3144019573014856794, 0.000000000000000000 ) ) ;
#2920=CARTESIAN_POINT ( 'NONE',  ( 3.533549941398215211, -54.99147314093924166, 0.1611374604154752754 ) ) ;
#2922=CARTESIAN_POINT ( 'NONE',  ( -1.180326523133921945, -55.13093161118004559, 0.1348352173942452270 ) ) ;
#2925=ORIENTED_EDGE ( 'NONE', *, *, #7382, .F. ) ;
#2928=AXIS2_PLACEMENT_3D ( 'NONE', #1806, #4101, #3539 ) ;
#2932=CIRCLE ( 'NONE', #1616, 0.9999999999999998890 ) ;
#2933=APPLICATION_CONTEXT ( 'automotive_design' ) ;
#2935=CARTESIAN_POINT ( 'NONE',  ( -3.235261603508409856, -66.01500717273368934, 1.164464255201294929 ) ) ;
#2936=DIRECTION ( 'NONE',  ( 0.3144019573014853464, -0.9492899500389726519, -7.355227538141627568E-16 ) ) ;
#2938=CARTESIAN_POINT ( 'NONE',  ( -4.248468832057555211, -63.21868707083201855, -2.033638508047526550 ) ) ;
#2941=CARTESIAN_POINT ( 'NONE',  ( 5.770703635693222644, -59.55204183230187454, 0.5638254346361636360 ) ) ;
#2942=CARTESIAN_POINT ( 'NONE',  ( 5.742131165818880056, -64.29439030986208081, -3.151051222873450630 ) ) ;
#2943=CARTESIAN_POINT ( 'NONE',  ( -15.08175531864075047, -33.99084820126180517, -5.041145139047909396 ) ) ;
#2945=CARTESIAN_POINT ( 'NONE',  ( -5.616612366066321194, -62.30416043735317544, 3.536847275893812537 ) ) ;
#2948=CARTESIAN_POINT ( 'NONE',  ( 4.689255334142830023, -62.66924379293478609, -1.721810340931042793 ) ) ;
#2949=CARTESIAN_POINT ( 'NONE',  ( 6.285636693253979779, -59.03245517747429716, 2.489777307435960374 ) ) ;
#2956=EDGE_CURVE ( 'NONE', #1033, #6355, #4994, .T. ) ;
#2959=CARTESIAN_POINT ( 'NONE',  ( -6.177019684192219806, -63.92521542081036756, -0.3671906505365997164 ) ) ;
#2971=CARTESIAN_POINT ( 'NONE',  ( 4.676675357529780364, -57.90541686953501710, 2.165367849443769810 ) ) ;
#2973=DIRECTION ( 'NONE',  ( 0.000000000000000000, 0.000000000000000000, 1.000000000000000000 ) ) ;
#2974=CARTESIAN_POINT ( 'NONE',  ( 4.690637055356551954, -57.05217919465406595, 0.4062669221328191749 ) ) ;
#2977=CARTESIAN_POINT ( 'NONE',  ( -5.063240685778024108, -62.12055065899711792, 3.262469527825359261 ) ) ;
#2979=CARTESIAN_POINT ( 'NONE',  ( -0.9970853242166300978, -65.67144495878099519, -1.280490079922569802 ) ) ;
#2980=CARTESIAN_POINT ( 'NONE',  ( 1.700848490796859958, -66.65813550864595527, 0.8993149516912349872 ) ) ;
#2981=DIRECTION ( 'NONE',  ( 0.2223191033124283789, 0.6712482523644727195, 0.7071067811865466846 ) ) ;
#2982=ORIENTED_EDGE ( 'NONE', *, *, #4996, .T. ) ;
#2987=DIRECTION ( 'NONE',  ( -0.9492883822130747662, 0.3144066910790599412, 0.000000000000000000 ) ) ;
#2988=CARTESIAN_POINT ( 'NONE',  ( -5.671911954242359499, -63.61502870002530585, -0.7222274751851948116 ) ) ;
#2994=CARTESIAN_POINT ( 'NONE',  ( 6.305975611789820690, -62.57522228252229723, -3.271841503593345024 ) ) ;
#2995=CARTESIAN_POINT ( 'NONE',  ( -6.239404450008960268, -62.05055862403510503, 1.429382062327010150 ) ) ;
#2999=CARTESIAN_POINT ( 'NONE',  ( -5.689067437457130616, -61.48253059702771850, 3.675478928603590489 ) ) ;
#3001=DIRECTION ( 'NONE',  ( -0.9492883822130744331, 0.3144066910790611624, 0.000000000000000000 ) ) ;
#3004=CARTESIAN_POINT ( 'NONE',  ( 4.061787823018702781, -64.57068682332180742, -1.219517233498399245 ) ) ;
#3007=CARTESIAN_POINT ( 'NONE',  ( 2.906897738665179975, -66.25564029441702019, 0.8681355557765302322 ) ) ;
#3009=VERTEX_POINT ( 'NONE', #3926 ) ;
#3010=CARTESIAN_POINT ( 'NONE',  ( -5.904042796847299712, -62.42803713013675093, 3.506543003539000392 ) ) ;
#3011=CIRCLE ( 'NONE', #6280, 2.500000000000000444 ) ;
#3014=CARTESIAN_POINT ( 'NONE',  ( -2.392055737067099841, -65.19778216667813808, -1.190937291917544050 ) ) ;
#3015=CARTESIAN_POINT ( 'NONE',  ( -6.097705871868670080, -61.85866295707492668, 3.539665806518350610 ) ) ;
#3021=CARTESIAN_POINT ( 'NONE',  ( -13.12502771320784056, -36.71825441132875767, 1.026284428608169819 ) ) ;
#3023=AXIS2_PLACEMENT_3D ( 'NONE', #4223, #3687, #1368 ) ;
#3025=CARTESIAN_POINT ( 'NONE',  ( 3.257640280419950241, -66.06664283717124420, -1.252360977842533751 ) ) ;
#3033=EDGE_CURVE ( 'NONE', #380, #1005, #511, .T. ) ;
#3034=CARTESIAN_POINT ( 'NONE',  ( -14.02739156872318027, -37.17434273187110705, -0.4662714048949997969 ) ) ;
#3035=CIRCLE ( 'NONE', #47, 1.000000000000000444 ) ;
#3036=FACE_OUTER_BOUND ( 'NONE', #3741, .T. ) ;
#3043=CARTESIAN_POINT ( 'NONE',  ( 1.397902174090916105, -65.57924198930768966, 0.6644065888002452791 ) ) ;
#3048=CARTESIAN_POINT ( 'NONE',  ( -2.599597233209017144, -55.21935138117550679, -2.163518569292217641 ) ) ;
#3049=CARTESIAN_POINT ( 'NONE',  ( -6.238986924797109701, -58.62463756020586914, -0.4569988612983747478 ) ) ;
#3053=EDGE_CURVE ( 'NONE', #210, #6757, #3035, .T. ) ;
#3057=CARTESIAN_POINT ( 'NONE',  ( 3.331090576803830139, -65.95739139720836874, 0.8111086825117052035 ) ) ;
#3058=CARTESIAN_POINT ( 'NONE',  ( 1.276103242900551882, -55.15251840166065733, -1.809563881513800876 ) ) ;
#3059=CARTESIAN_POINT ( 'NONE',  ( 5.267626090836840191, -63.86700364562991439, -1.442031773567929775 ) ) ;
#3061=ORIENTED_EDGE ( 'NONE', *, *, #4996, .F. ) ;
#3063=ORIENTED_EDGE ( 'NONE', *, *, #3053, .T. ) ;
#3066=CARTESIAN_POINT ( 'NONE',  ( -5.310432382237169513, -59.25281681403794209, -2.339912608914485936 ) ) ;
#3068=ORIENTED_EDGE ( 'NONE', *, *, #2334, .F. ) ;
#3072=CARTESIAN_POINT ( 'NONE',  ( 4.747874937083381930, -62.01186481602808698, -2.352241412846060697 ) ) ;
#3073=CARTESIAN_POINT ( 'NONE',  ( 1.316624512147740012, -66.75104842734066324, 3.019790780136459851 ) ) ;
#3078=CARTESIAN_POINT ( 'NONE',  ( -5.211262431554310126, -59.36811747016641050, -0.7503612693867500738 ) ) ;
#3079=DIRECTION ( 'NONE',  ( 0.3128416502900970286, -0.9445788350777319931, 0.09950339776592319330 ) ) ;
#3080=DIRECTION ( 'NONE',  ( 1.000000000000000000, 0.000000000000000000, 0.000000000000000000 ) ) ;
#3081=CARTESIAN_POINT ( 'NONE',  ( -4.642435027186547103, -56.98634068404612663, -2.320710962605212480 ) ) ;
#3082=EDGE_CURVE ( 'NONE', #6872, #380, #4135, .T. ) ;
#3083=ORIENTED_EDGE ( 'NONE', *, *, #3785, .F. ) ;
#3084=DIRECTION ( 'NONE',  ( 0.3128416502900970286, -0.9445788350777319931, 0.09950339776592319330 ) ) ;
#3087=CARTESIAN_POINT ( 'NONE',  ( -5.524241737545620090, -57.12730840725460979, 1.694319224817255165 ) ) ;
#3088=CARTESIAN_POINT ( 'NONE',  ( -6.026198395890769888, -63.94474587426248036, 1.222360836057740041 ) ) ;
#3096=CARTESIAN_POINT ( 'NONE',  ( -1.110895189285712181, -65.77251424999820983, -2.870029284013874360 ) ) ;
#3097=CARTESIAN_POINT ( 'NONE',  ( 1.878435065497310541, -54.43101827334665899, 2.142267462834059888 ) ) ;
#3101=ORIENTED_EDGE ( 'NONE', *, *, #1900, .F. ) ;
#3105=CARTESIAN_POINT ( 'NONE',  ( -6.129265975028279634, -62.42766041111902098, -0.6909925287373350766 ) ) ;
#3106=ORIENTED_EDGE ( 'NONE', *, *, #303, .F. ) ;
#3111=CARTESIAN_POINT ( 'NONE',  ( 1.275220786007323914, -54.66846601681689322, 0.1350250863793004130 ) ) ;
#3114=CARTESIAN_POINT ( 'NONE',  ( -6.322565549722802380, -62.54715718787130641, 3.405899984212338971 ) ) ;
#3115=CARTESIAN_POINT ( 'NONE',  ( -5.789985532050487826, -60.41058001130513588, -0.4326874901607719592 ) ) ;
#3116=ORIENTED_EDGE ( 'NONE', *, *, #2475, .T. ) ;
#3117=CARTESIAN_POINT ( 'NONE',  ( -14.41480805056212056, -36.00459628421619840, -4.334038357861370372 ) ) ;
#3123=CARTESIAN_POINT ( 'NONE',  ( -5.895051854024569771, -62.45358532148892294, 3.505907163650189950 ) ) ;
#3124=CARTESIAN_POINT ( 'NONE',  ( -2.038541806680159940, -53.77797276486428046, -0.2805255711276150588 ) ) ;
#3125=CARTESIAN_POINT ( 'NONE',  ( 15.08188723176695056, -33.99092340910145538, 5.072392329257909616 ) ) ;
#3131=LINE ( 'NONE', #2580, #6533 ) ;
#3132=CARTESIAN_POINT ( 'NONE',  ( 1.597826897138040048, -55.24069855439622501, 0.3109211183784004184 ) ) ;
#3134=CARTESIAN_POINT ( 'NONE',  ( -5.977281909777053315, -62.42932436707042854, 1.407931773894181227 ) ) ;
#3138=CIRCLE ( 'NONE', #5082, 1.000000000000000000 ) ;
#3140=ADVANCED_FACE ( 'NONE', ( #5113 ), #6654, .T. ) ;
#3146=CARTESIAN_POINT ( 'NONE',  ( 5.854317997614909785, -64.22630450538810010, 2.635376777014039718 ) ) ;
#3151=CARTESIAN_POINT ( 'NONE',  ( -9.311346830843410416, -51.41373841511902043, 2.533728595105000370 ) ) ;
#3153=CARTESIAN_POINT ( 'NONE',  ( -3.222464925939095171, -55.48519077065235194, -0.1302151132178846482 ) ) ;
#3155=EDGE_LOOP ( 'NONE', ( #5748, #6128, #5756, #5965, #4199, #2111 ) ) ;
#3158=DIRECTION ( 'NONE',  ( -1.602374898470634869E-16, 1.442524254523139935E-17, 1.000000000000000000 ) ) ;
#3159=CARTESIAN_POINT ( 'NONE',  ( -2.726528979675269859, -65.60628988660214134, -2.897654743900204721 ) ) ;
#3162=AXIS2_PLACEMENT_3D ( 'NONE', #3505, #4155, #3577 ) ;
#3165=CYLINDRICAL_SURFACE ( 'NONE', #3276, 0.9999999999999998890 ) ;
#3166=CARTESIAN_POINT ( 'NONE',  ( 5.267626090836840191, -63.86700364562991439, -1.442031773567929775 ) ) ;
#3168=CARTESIAN_POINT ( 'NONE',  ( 1.455885123031280148, -67.63619251397972221, 2.328451870335179752 ) ) ;
#3169=CYLINDRICAL_SURFACE ( 'NONE', #1698, 1.000000000000000888 ) ;
#3171=VERTEX_POINT ( 'NONE', #1227 ) ;
#3172=VERTEX_POINT ( 'NONE', #616 ) ;
#3173=DIRECTION ( 'NONE',  ( 0.000000000000000000, 0.000000000000000000, 1.000000000000000000 ) ) ;
#3175=CARTESIAN_POINT ( 'NONE',  ( -3.096824821213254975, -64.92072129780139278, 1.460348123614904514 ) ) ;
#3177=CARTESIAN_POINT ( 'NONE',  ( -3.758252532389416256, -55.38071557709576354, 1.827664687072033889 ) ) ;
#3181=EDGE_LOOP ( 'NONE', ( #5071, #311, #5954, #5446, #3068, #5989 ) ) ;
#3186=CARTESIAN_POINT ( 'NONE',  ( -2.887726905928315269, -66.20272978495717098, -0.9560320787877147897 ) ) ;
#3191=CARTESIAN_POINT ( 'NONE',  ( -5.996378862946620814, -62.15612413928192836, 3.522786485084270058 ) ) ;
#3192=ORIENTED_EDGE ( 'NONE', *, *, #2406, .T. ) ;
#3193=DIRECTION ( 'NONE',  ( -0.08966155106958693943, -0.9959722919136836383, 0.000000000000000000 ) ) ;
#3202=CARTESIAN_POINT ( 'NONE',  ( -8.408982975328068932, -50.95765009457664974, 2.526284428608170263 ) ) ;
#3204=CARTESIAN_POINT ( 'NONE',  ( 5.693513582185560473, -64.15546253253084785, -1.561391656022143914 ) ) ;
#3211=CARTESIAN_POINT ( 'NONE',  ( 1.985288149635364929, -66.63130641047898450, -3.284835754603986580 ) ) ;
#3213=CARTESIAN_POINT ( 'NONE',  ( -1.036475255397104833, -54.28545530925913454, 1.984742741622252948 ) ) ;
#3220=DIRECTION ( 'NONE',  ( 0.3128463504745289669, 0.9445772445362837777, 0.09950371902099817978 ) ) ;
#3222=CARTESIAN_POINT ( 'NONE',  ( 3.949972843796054178, -66.18831294452250802, -1.427832076542613793 ) ) ;
#3227=CARTESIAN_POINT ( 'NONE',  ( 2.986904076224405014, -66.15109244657664078, 2.931604786918900363 ) ) ;
#3232=EDGE_LOOP ( 'NONE', ( #2137, #773, #801, #4318, #3590, #5094 ) ) ;
#3233=CIRCLE ( 'NONE', #4011, 1.000000000000001776 ) ;
#3241=CARTESIAN_POINT ( 'NONE',  ( -3.551508372363994859, -54.02225908916108210, 1.181396430060940306 ) ) ;
#3242=DIRECTION ( 'NONE',  ( 0.3128463504745285229, 0.9445772445362839997, 0.09950371902099811039 ) ) ;
#3243=ORIENTED_EDGE ( 'NONE', *, *, #162, .T. ) ;
#3245=AXIS2_PLACEMENT_3D ( 'NONE', #4730, #2356, #6917 ) ;
#3248=CARTESIAN_POINT ( 'NONE',  ( 4.964513617332250384, -59.39532806039484569, 1.236961020452715054 ) ) ;
#3249=CARTESIAN_POINT ( 'NONE',  ( -9.358272925367041140, -51.27205205187813419, 2.526284428608170263 ) ) ;
#3250=CARTESIAN_POINT ( 'NONE',  ( -6.177096350592991669, -59.51804186297885479, 1.565423707298817080 ) ) ;
#3258=CARTESIAN_POINT ( 'NONE',  ( 5.904685685680689744, -64.36828453093134783, 1.045689304822035037 ) ) ;
#3263=CARTESIAN_POINT ( 'NONE',  ( -5.524241737545620090, -57.12730840725460979, 1.694319224817255165 ) ) ;
#3265=AXIS2_PLACEMENT_3D ( 'NONE', #1075, #2197, #1194 ) ;
#3270=ORIENTED_EDGE ( 'NONE', *, *, #3335, .T. ) ;
#3276=AXIS2_PLACEMENT_3D ( 'NONE', #5490, #2603, #4913 ) ;
#3279=CARTESIAN_POINT ( 'NONE',  ( 2.066956868921485224, -53.66058936408188629, 0.4281972772843347652 ) ) ;
#3282=ORIENTED_EDGE ( 'NONE', *, *, #6986, .F. ) ;
#3289=CARTESIAN_POINT ( 'NONE',  ( -4.559578989909869762, -57.69789612496867903, 1.459412177499654462 ) ) ;
#3292=CARTESIAN_POINT ( 'NONE',  ( -5.253023064401910247, -61.29850624113154822, 1.730934016304810363 ) ) ;
#3300=DIRECTION ( 'NONE',  ( 0.000000000000000000, 0.000000000000000000, 1.000000000000000000 ) ) ;
#3301=DIRECTION ( 'NONE',  ( -0.08966155106958693943, -0.9959722919136836383, 0.000000000000000000 ) ) ;
#3303=CARTESIAN_POINT ( 'NONE',  ( 6.144163068047750365, -64.45449589790229084, 2.063594979539779661 ) ) ;
#3308=CARTESIAN_POINT ( 'NONE',  ( 8.409045811045761099, -50.95764513735950629, -2.495037190209991707 ) ) ;
#3309=DIRECTION ( 'NONE',  ( 0.2223191033124284066, 0.6712482523644728305, 0.7071067811865467956 ) ) ;
#3314=CARTESIAN_POINT ( 'NONE',  ( -4.763494996734372933, -62.01236420069433564, 2.093068328189249261 ) ) ;
#3317=CARTESIAN_POINT ( 'NONE',  ( 3.193531232915834739, -66.77446787883670254, 1.223174286645849929 ) ) ;
#3319=ORIENTED_EDGE ( 'NONE', *, *, #3033, .T. ) ;
#3321=CARTESIAN_POINT ( 'NONE',  ( -4.816289696271150333, -61.50450503696147564, 2.285640538916479780 ) ) ;
#3326=CARTESIAN_POINT ( 'NONE',  ( -2.603817572988885054, -64.79915130424556935, -0.08835382460255962467 ) ) ;
#3335=EDGE_CURVE ( 'NONE', #3646, #5827, #4418, .T. ) ;
#3339=CARTESIAN_POINT ( 'NONE',  ( 7.003919171491410189, -62.62977488282763261, 1.976316849587809843 ) ) ;
#3345=CARTESIAN_POINT ( 'NONE',  ( -2.887726905928315269, -66.20272978495717098, -0.9560320787877147897 ) ) ;
#3346=EDGE_CURVE ( 'NONE', #1826, #5376, #982, .T. ) ;
#3349=CARTESIAN_POINT ( 'NONE',  ( -6.644288653247606646, -62.64468192876543640, 2.431384972305744796 ) ) ;
#3351=FACE_OUTER_BOUND ( 'NONE', #6500, .T. ) ;
#3352=CYLINDRICAL_SURFACE ( 'NONE', #2202, 1.000000000000000888 ) ;
#3354=CARTESIAN_POINT ( 'NONE',  ( 6.443572816261259995, -63.55558822192794111, -2.176462561484786118 ) ) ;
#3360=CARTESIAN_POINT ( 'NONE',  ( -4.847093383240289377, -61.94486680083809205, -1.943810276119404046 ) ) ;
#3363=CARTESIAN_POINT ( 'NONE',  ( -1.308638315835680022, -65.34704488060808103, -0.1780822347184347620 ) ) ;
#3365=CARTESIAN_POINT ( 'NONE',  ( -5.870834073365089445, -58.01445613662527734, -0.4538462669607478683 ) ) ;
#3369=AXIS2_PLACEMENT_3D ( 'NONE', #5142, #607, #6905 ) ;
#3375=CARTESIAN_POINT ( 'NONE',  ( -2.273841640848679901, -67.16083533941571204, 1.488471302465715018 ) ) ;
#3378=CARTESIAN_POINT ( 'NONE',  ( 5.695730293278450596, -62.33055481056936742, -2.502481404895003259 ) ) ;
#3393=CARTESIAN_POINT ( 'NONE',  ( -5.951685856498870386, -64.29772444222471961, -2.487703520802049262 ) ) ;
#3397=ORIENTED_EDGE ( 'NONE', *, *, #4416, .T. ) ;
#3400=CIRCLE ( 'NONE', #6765, 0.4999999999999918954 ) ;
#3403=CARTESIAN_POINT ( 'NONE',  ( -2.607408651135029842, -55.80429912246091106, 1.635486251833709881 ) ) ;
#3413=DIRECTION ( 'NONE',  ( 0.2223157560262047083, -0.6712493609847988152, 0.7071067811865449082 ) ) ;
#3417=CARTESIAN_POINT ( 'NONE',  ( -9.326988862351289100, -51.36650962737204651, 1.531247206272719374 ) ) ;
#3418=CARTESIAN_POINT ( 'NONE',  ( 1.894024985814124928, -67.53311321014548696, 0.2080693458549401353 ) ) ;
#3422=CARTESIAN_POINT ( 'NONE',  ( 14.97072768011073940, -34.32654753528365177, 2.597518595105000383 ) ) ;
#3425=EDGE_CURVE ( 'NONE', #6921, #4300, #5466, .T. ) ;
#3428=EDGE_LOOP ( 'NONE', ( #693, #2175 ) ) ;
#3434=CARTESIAN_POINT ( 'NONE',  ( 2.193175381750440245, -67.18695861934700986, -2.930484425198875087 ) ) ;
#3438=DIRECTION ( 'NONE',  ( -0.08966155106958693943, -0.9959722919136836383, 0.000000000000000000 ) ) ;
#3440=ADVANCED_FACE ( 'NONE', ( #5522 ), #3165, .T. ) ;
#3441=CARTESIAN_POINT ( 'NONE',  ( 5.164426235684419275, -63.32698789961681030, 0.7537993011490951023 ) ) ;
#3443=CARTESIAN_POINT ( 'NONE',  ( -14.63712380658832046, -35.33334692323139592, -3.626931576674818025 ) ) ;
#3444=ORIENTED_EDGE ( 'NONE', *, *, #4416, .F. ) ;
#3445=ORIENTED_EDGE ( 'NONE', *, *, #4170, .T. ) ;
#3451=CARTESIAN_POINT ( 'NONE',  ( 6.180415987647270626, -62.45112898858806716, 0.6030958204723052551 ) ) ;
#3453=CARTESIAN_POINT ( 'NONE',  ( 4.756074659365879143, -62.80135681555328375, -3.311393743080873975 ) ) ;
#3454=ORIENTED_EDGE ( 'NONE', *, *, #6726, .F. ) ;
#3455=ORIENTED_EDGE ( 'NONE', *, *, #6379, .F. ) ;
#3466=CARTESIAN_POINT ( 'NONE',  ( -0.004658654679648590799, -66.23339599434021352, 1.140748123765403355 ) ) ;
#3467=CARTESIAN_POINT ( 'NONE',  ( 6.272193759149150338, -58.74577472516177323, -1.694429590687548837 ) ) ;
#3470=CARTESIAN_POINT ( 'NONE',  ( -5.104186137876693508, -62.13399138291284629, 3.298500478949792480 ) ) ;
#3472=ADVANCED_FACE ( 'NONE', ( #6781 ), #3352, .T. ) ;
#3475=DIRECTION ( 'NONE',  ( -0.5224671166576538850, 0.8526594349512809368, 0.000000000000000000 ) ) ;
#3476=CARTESIAN_POINT ( 'NONE',  ( 4.348279337280104961, -63.27746244242579365, -1.677170969482009832 ) ) ;
#3478=CYLINDRICAL_SURFACE ( 'NONE', #5065, 0.9999999999999998890 ) ;
#3482=CARTESIAN_POINT ( 'NONE',  ( 14.02750760687355935, -37.17441268192290238, 0.4975185951050001831 ) ) ;
#3483=VERTEX_POINT ( 'NONE', #4042 ) ;
#3484=CARTESIAN_POINT ( 'NONE',  ( 6.071255580768259108, -56.77894568653594121, -1.427178034550365959 ) ) ;
#3486=CARTESIAN_POINT ( 'NONE',  ( -5.310432382237169513, -59.25281681403794209, -2.339912608914485936 ) ) ;
#3488=ORIENTED_EDGE ( 'NONE', *, *, #5324, .T. ) ;
#3490=CARTESIAN_POINT ( 'NONE',  ( -13.49899450467539985, -35.75040780681265318, -0.4662714048949997969 ) ) ;
#3491=AXIS2_PLACEMENT_3D ( 'NONE', #3443, #1195, #2385 ) ;
#3494=CARTESIAN_POINT ( 'NONE',  ( -6.216708800954390490, -58.75440211775612909, 1.606470739968075545 ) ) ;
#3497=EDGE_LOOP ( 'NONE', ( #66, #5282, #7173, #6764, #1328 ) ) ;
#3498=CARTESIAN_POINT ( 'NONE',  ( 2.576047814891095022, -64.81584722952422339, -0.4432308004904150223 ) ) ;
#3502=CARTESIAN_POINT ( 'NONE',  ( 5.544705546025709531, -62.26256661181761842, 0.7210154936787926960 ) ) ;
#3503=CARTESIAN_POINT ( 'NONE',  ( -5.982481740117790103, -62.36145600051965232, 1.442409191505919619 ) ) ;
#3505=CARTESIAN_POINT ( 'NONE',  ( -15.08175531864075047, -33.99084820126180517, -5.041145139047909396 ) ) ;
#3508=CARTESIAN_POINT ( 'NONE',  ( -5.094026379717228714, -62.13064902308300219, 3.289882701435055345 ) ) ;
#3513=CARTESIAN_POINT ( 'NONE',  ( -5.624257096981370552, -62.27449455720285698, -0.5715238816199899041 ) ) ;
#3515=CARTESIAN_POINT ( 'NONE',  ( -5.524241737545620090, -57.12730840725460979, 1.694319224817255165 ) ) ;
#3516=CARTESIAN_POINT ( 'NONE',  ( -14.49899450467539985, -35.75040780681265318, -2.566271404894997499 ) ) ;
#3525=CARTESIAN_POINT ( 'NONE',  ( -1.409024882572649906, -54.10038288851608712, -0.1041033434293599513 ) ) ;
#3533=B_SPLINE_CURVE_WITH_KNOTS ( 'NONE', 3,
 ( #6586, #3114, #6556, #907 ),
 .UNSPECIFIED., .F., .F.,
 ( 4, 4 ),
 ( 0.000000000000000000, 1.000000000000000000 ),
 .UNSPECIFIED. ) ;
#3536=LINE ( 'NONE', #2255, #4236 ) ;
#3539=DIRECTION ( 'NONE',  ( -0.3144019573014849023, 0.9492899500389726519, 0.000000000000000000 ) ) ;
#3540=CARTESIAN_POINT ( 'NONE',  ( 3.331090576803830139, -65.95739139720836874, 0.8111086825117052035 ) ) ;
#3546=ORIENTED_EDGE ( 'NONE', *, *, #1641, .F. ) ;
#3550=CARTESIAN_POINT ( 'NONE',  ( -5.076816837522959425, -57.40733507789485657, 1.813788655352380541 ) ) ;
#3551=CARTESIAN_POINT ( 'NONE',  ( -5.996378862946620814, -62.15612413928192836, 3.522786485084270058 ) ) ;
#3556=EDGE_CURVE ( 'NONE', #3706, #6490, #1373, .T. ) ;
#3560=CARTESIAN_POINT ( 'NONE',  ( 1.915558458284230214, -54.23376817553720031, 0.07315972318039029587 ) ) ;
#3568=CARTESIAN_POINT ( 'NONE',  ( 6.641713594241586804, -62.65488624492035541, -2.690269354371802368 ) ) ;
#3569=CARTESIAN_POINT ( 'NONE',  ( -5.996378862946620814, -62.15612413928192836, 3.522786485084270058 ) ) ;
#3570=CARTESIAN_POINT ( 'NONE',  ( -6.223557239263538321, -60.98460414740468138, 1.486641091859571162 ) ) ;
#3573=CARTESIAN_POINT ( 'NONE',  ( 1.277257345132870148, -65.35512402512885899, -0.3535023904437397113 ) ) ;
#3575=FACE_OUTER_BOUND ( 'NONE', #594, .T. ) ;
#3576=CARTESIAN_POINT ( 'NONE',  ( 0.8260371565349720058, -66.17440364758674320, -3.107556223232925241 ) ) ;
#3577=DIRECTION ( 'NONE',  ( -0.4328040977884316520, 0.5819352847797604200, 0.6884997728872834788 ) ) ;
#3582=UNCERTAINTY_MEASURE_WITH_UNIT (LENGTH_MEASURE( 1.000000000000000082E-05 ), #2815, 'distance_accuracy_value', 'NONE');
#3583=CARTESIAN_POINT ( 'NONE',  ( -1.556563313654149905, -55.35434594439572464, -0.3959639196582302456 ) ) ;
#3590=ORIENTED_EDGE ( 'NONE', *, *, #6211, .F. ) ;
#3593=CARTESIAN_POINT ( 'NONE',  ( 2.193175381750440245, -67.18695861934700986, -2.930484425198875087 ) ) ;
#3597=DIRECTION ( 'NONE',  ( 0.000000000000000000, 0.000000000000000000, 1.000000000000000000 ) ) ;
#3601=CARTESIAN_POINT ( 'NONE',  ( 6.061184043039538949, -62.50365188168748176, -3.430634321730453351 ) ) ;
#3607=CARTESIAN_POINT ( 'NONE',  ( 5.191094514348209898, -57.61090315545595786, 2.520404771314449732 ) ) ;
#3610=CARTESIAN_POINT ( 'NONE',  ( -5.408374332777167837, -58.11854958432094520, -2.399418114313899508 ) ) ;
#3616=DIRECTION ( 'NONE',  ( 0.3128463504745289669, 0.9445772445362837777, 0.09950371902099817978 ) ) ;
#3618=CARTESIAN_POINT ( 'NONE',  ( 6.187144687173720570, -58.64655194120005177, 0.3691021985165400809 ) ) ;
#3619=CARTESIAN_POINT ( 'NONE',  ( -4.780177894917470027, -57.84320307688069107, -2.250545046436859931 ) ) ;
#3620=CARTESIAN_POINT ( 'NONE',  ( 1.785462125252589960, -54.25404267560509908, 2.136629312307830375 ) ) ;
#3622=ADVANCED_FACE ( 'NONE', ( #87 ), #6253, .T. ) ;
#3630=CARTESIAN_POINT ( 'NONE',  ( -3.018293710664720297, -66.19764165108277609, -3.019563749174228207 ) ) ;
#3642=DIRECTION ( 'NONE',  ( 0.9492883822130744331, -0.3144066910790611624, 0.000000000000000000 ) ) ;
#3646=VERTEX_POINT ( 'NONE', #1219 ) ;
#3649=CARTESIAN_POINT ( 'NONE',  ( -5.065438427596520299, -62.07564176717611559, -0.9259012332463799622 ) ) ;
#3655=CARTESIAN_POINT ( 'NONE',  ( 0.9632665884170439341, -54.73762666295851886, -1.953671419500376816 ) ) ;
#3662=DIRECTION ( 'NONE',  ( 0.3144066910790610514, 0.9492883822130742111, 0.000000000000000000 ) ) ;
#3664=DIRECTION ( 'NONE',  ( 0.000000000000000000, 0.000000000000000000, 1.000000000000000000 ) ) ;
#3668=ADVANCED_FACE ( 'NONE', ( #3575 ), #5859, .T. ) ;
#3670=CARTESIAN_POINT ( 'NONE',  ( 5.271413390890690387, -61.79997272665566044, -1.279516964844005900 ) ) ;
#3677=CARTESIAN_POINT ( 'NONE',  ( -3.498019654714389581, -55.03494779767484602, -0.2490962732230048438 ) ) ;
#3678=ORIENTED_EDGE ( 'NONE', *, *, #4253, .F. ) ;
#3679=EDGE_CURVE ( 'NONE', #7067, #5349, #382, .T. ) ;
#3681=CARTESIAN_POINT ( 'NONE',  ( 5.768687865266859838, -59.13854474313614418, 2.609246528188839509 ) ) ;
#3684=CARTESIAN_POINT ( 'NONE',  ( 14.07443455944474131, -37.03272609524245240, -0.9950371902099899302 ) ) ;
#3687=DIRECTION ( 'NONE',  ( 0.9492899500389727629, 0.3144019573014849023, 0.000000000000000000 ) ) ;
#3690=CARTESIAN_POINT ( 'NONE',  ( -2.887726905928315269, -66.20272978495717098, -0.9560320787877147897 ) ) ;
#3692=CARTESIAN_POINT ( 'NONE',  ( 1.830733139179690161, -67.16965779809959258, 0.7798461408577649356 ) ) ;
#3693=CARTESIAN_POINT ( 'NONE',  ( -14.49899450467539985, -35.75040780681265318, -2.566271404894997499 ) ) ;
#3701=CARTESIAN_POINT ( 'NONE',  ( 5.944105978113960020, -62.47685828501489169, -3.593838583070729786 ) ) ;
#3702=CARTESIAN_POINT ( 'NONE',  ( 5.093888048015757342, -64.05487131086009356, 2.771559435373996738 ) ) ;
#3706=VERTEX_POINT ( 'NONE', #7074 ) ;
#3711=CARTESIAN_POINT ( 'NONE',  ( -1.735723365167664900, -67.19411771835910940, 0.9573769032209800134 ) ) ;
#3714=CARTESIAN_POINT ( 'NONE',  ( 3.069422284440780135, -65.49896014417400636, 0.9299900502622647780 ) ) ;
#3716=CYLINDRICAL_SURFACE ( 'NONE', #480, 1.000000000000001332 ) ;
#3717=CARTESIAN_POINT ( 'NONE',  ( -5.570007062648755891, -62.18452688224461866, -2.635462372538256215 ) ) ;
#3727=CARTESIAN_POINT ( 'NONE',  ( -6.728394430327000464, -62.68905628767773663, 2.815217869383099814 ) ) ;
#3738=CARTESIAN_POINT ( 'NONE',  ( -1.516811388151804829, -54.38796383586615235, 1.958561210572854483 ) ) ;
#3741=EDGE_LOOP ( 'NONE', ( #336, #5474, #3106, #519, #295, #2010 ) ) ;
#3742=TOROIDAL_SURFACE ( 'NONE', #743, 1.500000000000000000, 1.000000000000000000 ) ;
#3746=ADVANCED_FACE ( 'NONE', ( #1361 ), #3716, .T. ) ;
#3748=CARTESIAN_POINT ( 'NONE',  ( -3.132958547045754827, -66.67000521241658362, -1.075502346145061683 ) ) ;
#3755=CARTESIAN_POINT ( 'NONE',  ( -5.624257096981370552, -62.27449455720285698, -0.5715238816199899041 ) ) ;
#3756=AXIS2_PLACEMENT_3D ( 'NONE', #2012, #6722, #1010 ) ;
#3758=CIRCLE ( 'NONE', #7368, 1.000000000000000000 ) ;
#3760=CARTESIAN_POINT ( 'NONE',  ( -5.565225078471084608, -62.28720617293075179, 1.537195128485716378 ) ) ;
#3767=CARTESIAN_POINT ( 'NONE',  ( 5.676184037656430093, -63.13711808556965366, -1.485967351095627720 ) ) ;
#3770=CARTESIAN_POINT ( 'NONE',  ( 3.219971992657300053, -66.62470095071212484, 2.812725188592500203 ) ) ;
#3771=DIRECTION ( 'NONE',  ( 0.3144066910790613845, 0.9492883822130742111, 0.000000000000000000 ) ) ;
#3778=CARTESIAN_POINT ( 'NONE',  ( 2.671142801832544933, -55.70169962949673703, -1.720663637103989618 ) ) ;
#3780=CARTESIAN_POINT ( 'NONE',  ( 4.005285614311604903, -55.65094623700133525, 2.273239139415862198 ) ) ;
#3785=EDGE_CURVE ( 'NONE', #2328, #5405, #6001, .T. ) ;
#3788=DIRECTION ( 'NONE',  ( -0.2467992669038191755, 0.02032136184815236737, 0.9688535307818070264 ) ) ;
#3790=CARTESIAN_POINT ( 'NONE',  ( -6.599700898649300207, -61.96243991103532522, 3.420662994399620072 ) ) ;
#3793=EDGE_CURVE ( 'NONE', #232, #5405, #3533, .T. ) ;
#3795=CARTESIAN_POINT ( 'NONE',  ( -1.974098099753330171, -66.57628266072889289, 3.196874607719439876 ) ) ;
#3803=DIRECTION ( 'NONE',  ( -1.602374898470634869E-16, 1.442524254523139935E-17, 1.000000000000000000 ) ) ;
#3805=CARTESIAN_POINT ( 'NONE',  ( 6.472013764049630247, -56.98767972836586182, 1.711274884184114775 ) ) ;
#3807=ORIENTED_EDGE ( 'NONE', *, *, #6211, .T. ) ;
#3811=CARTESIAN_POINT ( 'NONE',  ( -2.708443266796834781, -56.15294253968003346, -1.503436295530243827 ) ) ;
#3813=CARTESIAN_POINT ( 'NONE',  ( 4.114990506629828459, -65.14581218975672527, 2.850248089031072407 ) ) ;
#3821=CARTESIAN_POINT ( 'NONE',  ( 6.187144687173720570, -58.64655194120005177, 0.3691021985165400809 ) ) ;
#3822=EDGE_CURVE ( 'NONE', #5827, #4944, #2869, .T. ) ;
#3826=CARTESIAN_POINT ( 'NONE',  ( -15.08175531864075047, -33.26559167236155190, -4.352666404962730162 ) ) ;
#3827=CARTESIAN_POINT ( 'NONE',  ( -6.097705871868670080, -61.85866295707492668, 3.539665806518350610 ) ) ;
#3832=CARTESIAN_POINT ( 'NONE',  ( -6.643389330756649613, -62.64438243220202196, 2.533637634891150459 ) ) ;
#3835=DIRECTION ( 'NONE',  ( 0.3144066910790611624, 0.9492883822130743221, 0.000000000000000000 ) ) ;
#3840=AXIS2_PLACEMENT_3D ( 'NONE', #2074, #983, #5597 ) ;
#3841=CARTESIAN_POINT ( 'NONE',  ( 3.914764119449064772, -54.23824460091720567, 1.533423736523834346 ) ) ;
#3848=CARTESIAN_POINT ( 'NONE',  ( 1.475197934039484071, -55.33068667649028782, 1.900472455802885818 ) ) ;
#3851=ORIENTED_EDGE ( 'NONE', *, *, #2406, .F. ) ;
#3852=CARTESIAN_POINT ( 'NONE',  ( 1.985288149635364929, -66.63130641047898450, -3.284835754603986580 ) ) ;
#3860=CARTESIAN_POINT ( 'NONE',  ( 6.751207790105429929, -62.61097121624884210, 0.9581327554396804613 ) ) ;
#3866=CARTESIAN_POINT ( 'NONE',  ( 3.660823140336725068, -65.74644859602665292, -1.309095517728299907 ) ) ;
#3870=AXIS2_PLACEMENT_3D ( 'NONE', #5132, #4600, #6255 ) ;
#3875=ADVANCED_FACE ( 'NONE', ( #425 ), #6118, .T. ) ;
#3882=CARTESIAN_POINT ( 'NONE',  ( 6.378760423371060639, -64.06988568591069111, -0.05691440262071967293 ) ) ;
#3884=AXIS2_PLACEMENT_3D ( 'NONE', #4503, #3242, #985 ) ;
#3889=CARTESIAN_POINT ( 'NONE',  ( -4.957894848432390589, -59.36360895465049481, -1.768545648133530879 ) ) ;
#3893=CARTESIAN_POINT ( 'NONE',  ( -4.930053471857299918, -61.64676491032937378, 0.1765652348176402209 ) ) ;
#3897=ORIENTED_EDGE ( 'NONE', *, *, #2035, .T. ) ;
#3901=EDGE_LOOP ( 'NONE', ( #3116, #1872, #4776, #5552, #2756, #2093 ) ) ;
#3905=CARTESIAN_POINT ( 'NONE',  ( 6.443572816261259995, -63.55558822192794111, -2.176462561484786118 ) ) ;
#3909=CARTESIAN_POINT ( 'NONE',  ( -5.563801105733269914, -63.69014839564722763, 1.341242183458755344 ) ) ;
#3920=CARTESIAN_POINT ( 'NONE',  ( -6.240992105565960735, -57.07993508854151798, -2.135104940435555765 ) ) ;
#3924=CARTESIAN_POINT ( 'NONE',  ( 4.922451174039159660, -61.67826628571419434, -0.7081498598146799273 ) ) ;
#3926=CARTESIAN_POINT ( 'NONE',  ( 10.26069562290071957, -51.72814510619807749, -2.502481404895003259 ) ) ;
#3927=CARTESIAN_POINT ( 'NONE',  ( -4.302337887170949671, -63.34626699285441020, 3.181678273100430054 ) ) ;
#3933=CARTESIAN_POINT ( 'NONE',  ( -3.018293710664720297, -66.19764165108277609, -3.019563749174228207 ) ) ;
#3942=CARTESIAN_POINT ( 'NONE',  ( 2.066956868921485224, -53.66058936408188629, 0.4281972772843347652 ) ) ;
#3943=ORIENTED_EDGE ( 'NONE', *, *, #38, .F. ) ;
#3947=DIRECTION ( 'NONE',  ( 0.3144019573014844582, -0.9492899500389728740, 0.000000000000000000 ) ) ;
#3949=DIRECTION ( 'NONE',  ( -1.602374898470634869E-16, 1.442524254523139935E-17, 1.000000000000000000 ) ) ;
#3950=CARTESIAN_POINT ( 'NONE',  ( 14.81352433457121975, -34.80119172639020064, 0.4975185951050001831 ) ) ;
#3957=CARTESIAN_POINT ( 'NONE',  ( 3.751014749966880224, -66.74975575182239140, 0.1208598729073953049 ) ) ;
#3962=CARTESIAN_POINT ( 'NONE',  ( 4.890810490072590611, -59.09042288871975757, -0.8837144134564199893 ) ) ;
#3966=DIRECTION ( 'NONE',  ( 0.9492899500389727629, 0.3144019573014849023, 0.000000000000000000 ) ) ;
#3967=CARTESIAN_POINT ( 'NONE',  ( 5.090297305459900556, -61.99464686763499088, 2.430409751936420282 ) ) ;
#3968=DIRECTION ( 'NONE',  ( 0.000000000000000000, -0.7252570966694443788, 0.6884781359858918037 ) ) ;
#3973=AXIS2_PLACEMENT_3D ( 'NONE', #2420, #5868, #7055 ) ;
#3980=AXIS2_PLACEMENT_3D ( 'NONE', #3125, #6527, #279 ) ;
#3982=CARTESIAN_POINT ( 'NONE',  ( -6.238287558858839787, -63.42668406018486849, 1.752565146537014895 ) ) ;
#3989=DIRECTION ( 'NONE',  ( -0.3144019573014849023, 0.9492899500389726519, 0.000000000000000000 ) ) ;
#3997=CIRCLE ( 'NONE', #5933, 2.499999999999996891 ) ;
#4000=CARTESIAN_POINT ( 'NONE',  ( 6.281284389406939894, -57.15453665621128465, 0.6930907858711948810 ) ) ;
#4003=CIRCLE ( 'NONE', #3265, 1.000000000000000000 ) ;
#4010=CARTESIAN_POINT ( 'NONE',  ( 5.175864525269250116, -61.68163375030346174, 0.3100344153189201202 ) ) ;
#4011=AXIS2_PLACEMENT_3D ( 'NONE', #2141, #2181, #1591 ) ;
#4018=ORIENTED_EDGE ( 'NONE', *, *, #707, .T. ) ;
#4022=DIRECTION ( 'NONE',  ( 0.3144066910790611624, 0.9492883822130743221, 0.000000000000000000 ) ) ;
#4027=CARTESIAN_POINT ( 'NONE',  ( -1.862703854971429873, -67.54117654042293850, 0.3860096597272351659 ) ) ;
#4028=ORIENTED_EDGE ( 'NONE', *, *, #3793, .T. ) ;
#4032=SURFACE_SIDE_STYLE ('',( #7370 ) ) ;
#4035=CARTESIAN_POINT ( 'NONE',  ( 5.564888630279786419, -62.34576501924355796, -3.501689517682560648 ) ) ;
#4038=EDGE_CURVE ( 'NONE', #6025, #6356, #458, .T. ) ;
#4040=VERTEX_POINT ( 'NONE', #2820 ) ;
#4042=CARTESIAN_POINT ( 'NONE',  ( -9.389556988382800284, -51.17759447638420767, 3.521321650943620707 ) ) ;
#4043=DIRECTION ( 'NONE',  ( 0.000000000000000000, -0.7252570966694443788, 0.6884781359858918037 ) ) ;
#4044=CARTESIAN_POINT ( 'NONE',  ( -6.814417183322500016, -58.48210382454914935, -0.1019614231452001113 ) ) ;
#4051=CARTESIAN_POINT ( 'NONE',  ( -5.065438427596520299, -62.07564176717611559, -0.9259012332463799622 ) ) ;
#4059=CARTESIAN_POINT ( 'NONE',  ( 5.396949887678069935, -64.06165292293543700, 0.6913201402231599069 ) ) ;
#4061=CARTESIAN_POINT ( 'NONE',  ( 4.826828241146579934, -57.92957641372471755, 0.5758163846279100717 ) ) ;
#4064=DIRECTION ( 'NONE',  ( -0.9492883822130744331, 0.3144066910790611624, 0.000000000000000000 ) ) ;
#4081=CARTESIAN_POINT ( 'NONE',  ( -1.747150726250749964, -54.79256248330700174, -0.04158717877314997702 ) ) ;
#4083=CARTESIAN_POINT ( 'NONE',  ( 3.059030343303239974, -54.77303090793805040, 0.1039292770420399137 ) ) ;
#4086=EDGE_LOOP ( 'NONE', ( #3897, #4479, #4400, #6121, #2534, #1971 ) ) ;
#4091=CARTESIAN_POINT ( 'NONE',  ( -5.982481740117790103, -62.36145600051965232, 1.442409191505919619 ) ) ;
#4092=CARTESIAN_POINT ( 'NONE',  ( 15.02372294165784794, -37.34713278632150235, -0.9950371902099899302 ) ) ;
#4101=DIRECTION ( 'NONE',  ( 0.9492899500389727629, 0.3144019573014849023, 0.000000000000000000 ) ) ;
#4102=CARTESIAN_POINT ( 'NONE',  ( -3.156642594714314853, -54.82761582543010093, 1.871643660998590697 ) ) ;
#4106=CARTESIAN_POINT ( 'NONE',  ( -1.429016193381374089, -55.57463605963037168, -1.413872718151093721 ) ) ;
#4109=CARTESIAN_POINT ( 'NONE',  ( -3.697637789055789881, -65.78881948023087034, 1.221121406208630411 ) ) ;
#4120=CARTESIAN_POINT ( 'NONE',  ( 4.638831626566389588, -63.05209213275327329, 0.3994218305236152400 ) ) ;
#4121=CARTESIAN_POINT ( 'NONE',  ( 5.619938529503549773, -63.59344562873818774, 0.6343307546824898946 ) ) ;
#4122=FACE_OUTER_BOUND ( 'NONE', #6873, .T. ) ;
#4123=COLOUR_RGB ( '', 0.72549020, 0.75294118, 0.79215686) ;
#4127=ORIENTED_EDGE ( 'NONE', *, *, #3082, .F. ) ;
#4133=CARTESIAN_POINT ( 'NONE',  ( -6.921793923077749433, -58.90709844370859116, -2.222636374480685184 ) ) ;
#4135=CIRCLE ( 'NONE', #880, 1.000000000000001110 ) ;
#4144=TOROIDAL_SURFACE ( 'NONE', #4987, 1.500000000000000000, 1.000000000000000000 ) ;
#4147=CARTESIAN_POINT ( 'NONE',  ( -0.9369902355999032428, -66.67870154919400250, 1.040922737850055846 ) ) ;
#4148=ORIENTED_EDGE ( 'NONE', *, *, #3793, .F. ) ;
#4149=AXIS2_PLACEMENT_3D ( 'NONE', #2662, #2549, #3788 ) ;
#4150=CARTESIAN_POINT ( 'NONE',  ( -9.311346830843410416, -51.41373841511900622, 1.033728595105000148 ) ) ;
#4154=CARTESIAN_POINT ( 'NONE',  ( -3.079777581550224852, -54.72070545288789134, -0.1918259013367045740 ) ) ;
#4155=DIRECTION ( 'NONE',  ( 0.2223157560262044585, -0.6712493609847989262, 0.7071067811865449082 ) ) ;
#4161=ADVANCED_FACE ( 'NONE', ( #2402 ), #5256, .T. ) ;
#4162=CARTESIAN_POINT ( 'NONE',  ( 1.570963842414029976, -66.14661321919228953, 1.018783762524700265 ) ) ;
#4170=EDGE_CURVE ( 'NONE', #3172, #477, #6610, .T. ) ;
#4172=CARTESIAN_POINT ( 'NONE',  ( 6.202282335592980367, -63.50128988325390367, -3.194577187992014622 ) ) ;
#4174=VERTEX_POINT ( 'NONE', #7195 ) ;
#4177=CARTESIAN_POINT ( 'NONE',  ( 9.311407240687648468, -51.41373841511900622, -2.502481404895003259 ) ) ;
#4183=CARTESIAN_POINT ( 'NONE',  ( 4.638831626566389588, -63.05209213275327329, 0.3994218305236152400 ) ) ;
#4184=DIRECTION ( 'NONE',  ( -0.5224671166576538850, 0.8526594349512809368, 0.000000000000000000 ) ) ;
#4185=CARTESIAN_POINT ( 'NONE',  ( 4.670395546267172904, -63.95756402795250750, -3.369593122188990542 ) ) ;
#4188=FACE_OUTER_BOUND ( 'NONE', #3232, .T. ) ;
#4191=CARTESIAN_POINT ( 'NONE',  ( -2.585448123472324777, -55.65377943239024461, 0.04593497335228470535 ) ) ;
#4199=ORIENTED_EDGE ( 'NONE', *, *, #4521, .F. ) ;
#4202=CARTESIAN_POINT ( 'NONE',  ( 5.674632694949170109, -63.26545500802649258, -3.549449971387770297 ) ) ;
#4208=EDGE_CURVE ( 'NONE', #1675, #3009, #4341, .T. ) ;
#4211=CARTESIAN_POINT ( 'NONE',  ( -14.97059744062764075, -34.32647288175419931, -2.566271404895000163 ) ) ;
#4214=CARTESIAN_POINT ( 'NONE',  ( -1.974098099753330171, -66.57628266072889289, 3.196874607719439876 ) ) ;
#4217=CARTESIAN_POINT ( 'NONE',  ( 14.18471095241310032, -36.69976849081635351, 2.597518595105000383 ) ) ;
#4218=CARTESIAN_POINT ( 'NONE',  ( 3.023925381325990092, -64.82443887782423531, -1.545558412227113765 ) ) ;
#4221=CARTESIAN_POINT ( 'NONE',  ( 5.790058697650237285, -60.49223513209997094, -1.481755374152989191 ) ) ;
#4223=CARTESIAN_POINT ( 'NONE',  ( -9.311346830843410416, -51.41373841511900622, 1.033728595105000148 ) ) ;
#4227=CARTESIAN_POINT ( 'NONE',  ( -6.216708800954390490, -58.75440211775612909, 1.606470739968075545 ) ) ;
#4234=LINE ( 'NONE', #3021, #4736 ) ;
#4235=CIRCLE ( 'NONE', #7357, 0.4999999999999991118 ) ;
#4236=VECTOR ( 'NONE', #2335, 1000.000000000000000 ) ;
#4238=CARTESIAN_POINT ( 'NONE',  ( 4.666229687490379696, -57.64092629874981810, -1.544454925248829991 ) ) ;
#4240=EDGE_CURVE ( 'NONE', #5842, #1750, #1435, .T. ) ;
#4244=VERTEX_POINT ( 'NONE', #6674 ) ;
#4251=CARTESIAN_POINT ( 'NONE',  ( 5.642462292687943304, -62.26538107922269205, -1.493771565540467305 ) ) ;
#4252=CARTESIAN_POINT ( 'NONE',  ( 3.219971992657300053, -66.62470095071212484, 2.812725188592500203 ) ) ;
#4253=EDGE_CURVE ( 'NONE', #7181, #5827, #4330, .T. ) ;
#4258=CARTESIAN_POINT ( 'NONE',  ( -1.241878142352246028, -55.26848170174031338, 1.724521099399885182 ) ) ;
#4259=AXIS2_PLACEMENT_3D ( 'NONE', #2943, #6417, #1262 ) ;
#4261=CARTESIAN_POINT ( 'NONE',  ( 14.49911764349215915, -35.75048010860329839, 0.4975185951050001831 ) ) ;
#4265=CARTESIAN_POINT ( 'NONE',  ( 0.06232375252353471867, -54.65437704685372466, -2.006095305823016428 ) ) ;
#4269=DIRECTION ( 'NONE',  ( 0.1860016876085203441, -0.1636620475539279917, 0.9688230521603200529 ) ) ;
#4273=CARTESIAN_POINT ( 'NONE',  ( 1.700848490796859958, -66.65813550864595527, 0.8993149516912349872 ) ) ;
#4274=CARTESIAN_POINT ( 'NONE',  ( 5.854317997614909785, -64.22630450538810010, 2.635376777014039718 ) ) ;
#4276=ORIENTED_EDGE ( 'NONE', *, *, #7286, .T. ) ;
#4281=CARTESIAN_POINT ( 'NONE',  ( -4.739687333205909958, -61.73825078254577647, 2.268939929871689909 ) ) ;
#4282=CARTESIAN_POINT ( 'NONE',  ( -5.737183749403212296, -62.91840231736271960, 3.479437450128457954 ) ) ;
#4285=ORIENTED_EDGE ( 'NONE', *, *, #6428, .T. ) ;
#4291=CARTESIAN_POINT ( 'NONE',  ( 1.830733139179690161, -67.16965779809959258, 0.7798461408577649356 ) ) ;
#4293=ORIENTED_EDGE ( 'NONE', *, *, #3556, .T. ) ;
#4294=EDGE_CURVE ( 'NONE', #4944, #4040, #3233, .T. ) ;
#4296=CARTESIAN_POINT ( 'NONE',  ( 5.677676720488819662, -58.78440004686129328, 0.4885712913175552785 ) ) ;
#4297=FACE_OUTER_BOUND ( 'NONE', #5877, .T. ) ;
#4299=CARTESIAN_POINT ( 'NONE',  ( -2.621169780003727467, -55.22978393027467803, -0.06561799439619847574 ) ) ;
#4300=VERTEX_POINT ( 'NONE', #3202 ) ;
#4306=CARTESIAN_POINT ( 'NONE',  ( 6.162074140922939591, -62.32076522084695114, 2.666565443060120444 ) ) ;
#4307=CARTESIAN_POINT ( 'NONE',  ( -6.841972559203830961, -62.34857902771452842, 2.832214187714990228 ) ) ;
#4308=FACE_OUTER_BOUND ( 'NONE', #6607, .T. ) ;
#4309=EDGE_LOOP ( 'NONE', ( #3192, #2842, #2201, #2732, #2277, #3546 ) ) ;
#4315=CARTESIAN_POINT ( 'NONE',  ( -4.892892059336399591, -61.27075929137718191, 2.302341147961269652 ) ) ;
#4316=DIRECTION ( 'NONE',  ( 0.3128416502900965290, -0.9445788350777319931, 0.09950339776592478924 ) ) ;
#4317=CARTESIAN_POINT ( 'NONE',  ( 5.012342441489318290, -56.71631922511256363, 2.351956307816288394 ) ) ;
#4318=ORIENTED_EDGE ( 'NONE', *, *, #1132, .T. ) ;
#4322=CARTESIAN_POINT ( 'NONE',  ( 14.07443455944474131, -37.03272609524245240, -0.9950371902099899302 ) ) ;
#4324=CARTESIAN_POINT ( 'NONE',  ( 1.402950248545461909, -54.15620739517822813, 0.01614447287717020105 ) ) ;
#4325=ORIENTED_EDGE ( 'NONE', *, *, #5421, .F. ) ;
#4329=CARTESIAN_POINT ( 'NONE',  ( -2.607408651135029842, -55.80429912246091106, 1.635486251833709881 ) ) ;
#4330=CIRCLE ( 'NONE', #6026, 1.000000000000001776 ) ;
#4331=ORIENTED_EDGE ( 'NONE', *, *, #3556, .F. ) ;
#4336=ORIENTED_EDGE ( 'NONE', *, *, #1363, .T. ) ;
#4338=CIRCLE ( 'NONE', #3491, 1.000000000000000888 ) ;
#4341=LINE ( 'NONE', #6629, #4451 ) ;
#4343=CARTESIAN_POINT ( 'NONE',  ( 5.919885402076849878, -56.76393675504415626, 0.1623732496884200682 ) ) ;
#4351=CARTESIAN_POINT ( 'NONE',  ( 0.9735761768007340500, -65.42433328568066031, 1.767115439505955177 ) ) ;
#4354=CARTESIAN_POINT ( 'NONE',  ( -3.638963596321122651, -65.59027719068511431, 3.295737659246797957 ) ) ;
#4356=CARTESIAN_POINT ( 'NONE',  ( 4.520351875826989385, -63.47384446676466752, 0.9302720625520102260 ) ) ;
#4361=CIRCLE ( 'NONE', #2666, 0.9999999999999998890 ) ;
#4362=( NAMED_UNIT ( * ) SI_UNIT ( $, .STERADIAN. ) SOLID_ANGLE_UNIT ( ) );
#4366=CARTESIAN_POINT ( 'NONE',  ( 5.919885402076849878, -56.76393675504415626, 0.1623732496884200682 ) ) ;
#4370=ORIENTED_EDGE ( 'NONE', *, *, #6468, .T. ) ;
#4371=DIRECTION ( 'NONE',  ( 0.2223191033124284066, 0.6712482523644728305, 0.7071067811865466846 ) ) ;
#4373=CARTESIAN_POINT ( 'NONE',  ( -5.354034084503060065, -64.02545556441495478, -0.7792797212839647214 ) ) ;
#4376=CARTESIAN_POINT ( 'NONE',  ( -10.26063678088237907, -51.72814037242050489, 2.533728595105000370 ) ) ;
#4385=DIRECTION ( 'NONE',  ( -0.08966155106958693943, -0.9959722919136836383, 0.000000000000000000 ) ) ;
#4388=CARTESIAN_POINT ( 'NONE',  ( -6.177752788274950113, -57.21669580536380550, -0.5454192084659099660 ) ) ;
#4392=ADVANCED_FACE ( 'NONE', ( #6158 ), #7332, .T. ) ;
#4395=CARTESIAN_POINT ( 'NONE',  ( -2.954381708604445045, -64.87272166844897470, 3.050067095118260241 ) ) ;
#4397=CARTESIAN_POINT ( 'NONE',  ( 6.229763166278965869, -60.90327177492465438, 0.4901581683790414701 ) ) ;
#4400=ORIENTED_EDGE ( 'NONE', *, *, #7152, .F. ) ;
#4401=ORIENTED_EDGE ( 'NONE', *, *, #7328, .T. ) ;
#4404=DIRECTION ( 'NONE',  ( 0.3144019573014847913, -0.9492899500389727629, 0.000000000000000000 ) ) ;
#4407=CARTESIAN_POINT ( 'NONE',  ( 1.414957918137925930, -67.26958221326191278, 2.900267041832249593 ) ) ;
#4411=CARTESIAN_POINT ( 'NONE',  ( 5.416018991692120643, -63.93240027730202968, 2.754852738177090643 ) ) ;
#4414=B_SPLINE_CURVE_WITH_KNOTS ( 'NONE', 3,
 ( #808, #4282, #2008, #5533, #4926, #4354, #6134, #6606, #6102, #2540, #6645, #2617, #3813, #1492, #3702, #2403, #4714, #2090, #839, #4847, #4317, #5885, #3780, #6997, #3097, #1842, #5503, #3213, #3738, #1447, #3177, #4959, #926, #3250, #361, #3570, #3134, #887, #1290, #326, #7208, #6021, #4147, #7246, #6444, #5453, #2044, #1970, #290, #2652, #7136, #4397, #6685, #959, #1527, #2584, #5413, #247, #113, #4890, #6573, #1413, #7171, #6063, #402, #999, #7279, #3365, #1116, #1639, #7353, #1076, #2836, #1673, #1160, #4547, #1561, #1041, #6242, #6717, #5677, #2273, #1607, #2118, #5153 ),
 .UNSPECIFIED., .F., .F.,
 ( 4, 2, 2, 1, 2, 2, 2, 2, 2, 2, 1, 2, 2, 2, 2, 2, 2, 1, 2, 2, 2, 2, 1, 2, 2, 2, 2, 2, 2, 1, 2, 2, 2, 2, 2, 2, 1, 2, 2, 2, 2, 2, 2, 1, 2, 4 ),
 ( 0.000000000000000000, 0.01562500000000017347, 0.03125000000000034694, 0.06250000000000038858, 0.07812500000000047184, 0.09375000000000056899, 0.1250000000000006661, 0.1406250000000005829, 0.1562500000000004996, 0.1875000000000007772, 0.2187500000000010270, 0.2343750000000011657, 0.2500000000000012768, 0.2812500000000013878, 0.2968750000000014433, 0.3125000000000014988, 0.3437500000000017208, 0.3750000000000018874, 0.3906250000000019429, 0.4062500000000019984, 0.4375000000000021649, 0.4531250000000021094, 0.4687500000000019984, 0.5000000000000017764, 0.5312500000000016653, 0.5468750000000017764, 0.5625000000000017764, 0.5937500000000017764, 0.6093750000000017764, 0.6250000000000016653, 0.6562500000000015543, 0.6875000000000013323, 0.7031250000000012212, 0.7187500000000012212, 0.7500000000000009992, 0.7656250000000009992, 0.7812500000000008882, 0.8125000000000007772, 0.8437500000000006661, 0.8593750000000005551, 0.8750000000000003331, 0.9062500000000003331, 0.9218750000000002220, 0.9375000000000002220, 0.9687500000000001110, 1.000000000000000000 ),
 .UNSPECIFIED. ) ;
#4416=EDGE_CURVE ( 'NONE', #7272, #3172, #2895, .T. ) ;
#4418=LINE ( 'NONE', #1548, #4743 ) ;
#4421=CARTESIAN_POINT ( 'NONE',  ( -6.362523631248359735, -64.09785492953841413, 0.6509934082767404595 ) ) ;
#4426=CARTESIAN_POINT ( 'NONE',  ( 9.311407240687648468, -51.41373841511902043, -1.002481404894999928 ) ) ;
#4427=CARTESIAN_POINT ( 'NONE',  ( 1.576955190785845007, -65.26733347271304808, -2.474060432887700500 ) ) ;
#4436=CARTESIAN_POINT ( 'NONE',  ( -14.49899450467539985, -35.75040780681265318, -2.566271404894997499 ) ) ;
#4438=CARTESIAN_POINT ( 'NONE',  ( -6.994430249510970476, -62.66069223349322925, -1.382237850844937777 ) ) ;
#4445=CARTESIAN_POINT ( 'NONE',  ( -3.235261603508409856, -66.01500717273368934, 1.164464255201294929 ) ) ;
#4451=VECTOR ( 'NONE', #3662, 1000.000000000000227 ) ;
#4456=CARTESIAN_POINT ( 'NONE',  ( 3.455862201155819768, -54.25194821296495462, -1.605226101400722083 ) ) ;
#4461=CARTESIAN_POINT ( 'NONE',  ( 0.9735761768007340500, -65.42433328568066031, 1.767115439505955177 ) ) ;
#4464=CARTESIAN_POINT ( 'NONE',  ( -5.155987128177820900, -61.76400128369626685, 1.194474120832875519 ) ) ;
#4468=ORIENTED_EDGE ( 'NONE', *, *, #943, .T. ) ;
#4473=EDGE_CURVE ( 'NONE', #4852, #4770, #5059, .T. ) ;
#4477=CARTESIAN_POINT ( 'NONE',  ( -6.362523631248359735, -64.09785492953841413, 0.6509934082767404595 ) ) ;
#4479=ORIENTED_EDGE ( 'NONE', *, *, #7190, .T. ) ;
#4484=CARTESIAN_POINT ( 'NONE',  ( -5.628700163094269016, -63.23550210468251009, 3.461537593744290042 ) ) ;
#4500=CARTESIAN_POINT ( 'NONE',  ( 14.49911764349215915, -35.75048010860329839, 2.597518595105000383 ) ) ;
#4502=CARTESIAN_POINT ( 'NONE',  ( 1.894024985814124928, -67.53311321014548696, 0.2080693458549401353 ) ) ;
#4503=CARTESIAN_POINT ( 'NONE',  ( 9.358334193258830425, -51.27205182843857045, -2.495037190209989930 ) ) ;
#4508=CARTESIAN_POINT ( 'NONE',  ( -4.461725341067024786, -62.58642870417541104, 2.208339520507450082 ) ) ;
#4509=CARTESIAN_POINT ( 'NONE',  ( 14.49911764349215915, -35.75048010860329839, 2.597518595105000383 ) ) ;
#4511=CARTESIAN_POINT ( 'NONE',  ( 2.735691016399460107, -56.17047939608508500, 0.9718516700694501687 ) ) ;
#4515=CARTESIAN_POINT ( 'NONE',  ( -4.450126406946254498, -63.33667035482537244, 1.592103300391294773 ) ) ;
#4519=ORIENTED_EDGE ( 'NONE', *, *, #1132, .F. ) ;
#4521=EDGE_CURVE ( 'NONE', #4770, #7318, #1327, .T. ) ;
#4524=CARTESIAN_POINT ( 'NONE',  ( 5.790006757277029514, -62.30949558554882373, -1.494673596136803839 ) ) ;
#4525=CARTESIAN_POINT ( 'NONE',  ( -1.424128410011220147, -67.64226375110297340, -1.734372748508781870 ) ) ;
#4526=CARTESIAN_POINT ( 'NONE',  ( -14.18459254737392072, -36.69969775685165558, -0.4662714048949997969 ) ) ;
#4527=CARTESIAN_POINT ( 'NONE',  ( -6.239404450008960268, -62.05055862403510503, 1.429382062327010150 ) ) ;
#4536=CARTESIAN_POINT ( 'NONE',  ( 3.575547067216904740, -66.56692562923595347, -0.8973241761454349152 ) ) ;
#4540=EDGE_CURVE ( 'NONE', #3706, #7067, #4874, .T. ) ;
#4542=CARTESIAN_POINT ( 'NONE',  ( 5.193956696153660069, -59.28518064773341933, 2.254869812567109832 ) ) ;
#4543=DIRECTION ( 'NONE',  ( -1.602374898470634869E-16, 1.442524254523139935E-17, 1.000000000000000000 ) ) ;
#4545=CARTESIAN_POINT ( 'NONE',  ( -4.957894848432390589, -59.36360895465049481, -1.768545648133530879 ) ) ;
#4547=CARTESIAN_POINT ( 'NONE',  ( -2.865380587567759374, -66.05540079135724341, -0.9521156314410413879 ) ) ;
#4549=EDGE_CURVE ( 'NONE', #6356, #354, #2286, .T. ) ;
#4557=CARTESIAN_POINT ( 'NONE',  ( -6.268616217933410617, -56.62827303305337523, 1.003072567477500066 ) ) ;
#4560=ORIENTED_EDGE ( 'NONE', *, *, #4294, .F. ) ;
#4567=ORIENTED_EDGE ( 'NONE', *, *, #669, .T. ) ;
#4572=CARTESIAN_POINT ( 'NONE',  ( -3.381846796090564933, -54.21055914560344746, 0.1632119451740500493 ) ) ;
#4577=VECTOR ( 'NONE', #5822, 1000.000000000000114 ) ;
#4579=DIRECTION ( 'NONE',  ( 2.857391495672265093E-16, 4.793132013414519254E-17, 1.000000000000000000 ) ) ;
#4581=CARTESIAN_POINT ( 'NONE',  ( -5.725946002089390419, -61.92844332740136792, 1.548851071596535123 ) ) ;
#4583=DIRECTION ( 'NONE',  ( 0.3144066910790610514, 0.9492883822130742111, 0.000000000000000000 ) ) ;
#4586=ORIENTED_EDGE ( 'NONE', *, *, #6120, .F. ) ;
#4597=CARTESIAN_POINT ( 'NONE',  ( -6.733769393910259637, -61.90091566649680743, 1.831080987178660191 ) ) ;
#4600=DIRECTION ( 'NONE',  ( 0.3144066910790611624, 0.9492883822130744331, 6.800116025829053242E-16 ) ) ;
#4601=DIRECTION ( 'NONE',  ( -0.3144066910790611624, -0.9492883822130743221, 0.000000000000000000 ) ) ;
#4606=CIRCLE ( 'NONE', #1586, 1.000000000000000000 ) ;
#4608=AXIS2_PLACEMENT_3D ( 'NONE', #789, #2162, #7322 ) ;
#4609=DIRECTION ( 'NONE',  ( 0.3144066910790611624, 0.9492883822130744331, 0.000000000000000000 ) ) ;
#4613=CARTESIAN_POINT ( 'NONE',  ( -6.626722312431940765, -62.23055248060769884, 1.814117920127710226 ) ) ;
#4619=CARTESIAN_POINT ( 'NONE',  ( 9.311407240687648468, -51.41373841511902043, -1.502481404894999928 ) ) ;
#4623=AXIS2_PLACEMENT_3D ( 'NONE', #805, #2537, #177 ) ;
#4624=CARTESIAN_POINT ( 'NONE',  ( -14.49899450467539985, -35.75040780681265318, -2.566271404894997499 ) ) ;
#4625=CARTESIAN_POINT ( 'NONE',  ( -1.449391072403324099, -66.17791180637956927, 1.195139069250764852 ) ) ;
#4628=CYLINDRICAL_SURFACE ( 'NONE', #3245, 0.9999999999999980016 ) ;
#4638=CARTESIAN_POINT ( 'NONE',  ( 3.455862201155819768, -54.25194821296495462, -1.605226101400722083 ) ) ;
#4639=DIRECTION ( 'NONE',  ( 0.000000000000000000, -0.7252570966694443788, 0.6884781359858918037 ) ) ;
#4640=CARTESIAN_POINT ( 'NONE',  ( 1.662636012147085118, -65.62619303409478277, -3.045852711070930141 ) ) ;
#4651=ORIENTED_EDGE ( 'NONE', *, *, #6120, .T. ) ;
#4663=CARTESIAN_POINT ( 'NONE',  ( -5.101403815575769940, -63.43555091703197490, 1.460123530859765317 ) ) ;
#4665=DIRECTION ( 'NONE',  ( 0.3128416502900974727, -0.9445788350777317710, 0.09950339776592416474 ) ) ;
#4671=CARTESIAN_POINT ( 'NONE',  ( -1.794944750655344867, -54.19869589391355191, -2.224588173883939035 ) ) ;
#4673=ADVANCED_FACE ( 'NONE', ( #2104 ), #1581, .T. ) ;
#4676=CARTESIAN_POINT ( 'NONE',  ( -14.10560172626255948, -36.93819879313630139, 2.021321650943620263 ) ) ;
#4678=CARTESIAN_POINT ( 'NONE',  ( 6.162074140922939591, -62.32076522084695114, 2.666565443060120444 ) ) ;
#4679=EDGE_CURVE ( 'NONE', #5405, #3706, #5510, .T. ) ;
#4683=CARTESIAN_POINT ( 'NONE',  ( 4.964513617332250384, -59.39532806039484569, 1.236961020452715054 ) ) ;
#4684=CARTESIAN_POINT ( 'NONE',  ( -14.49899450467539985, -35.75040780681265318, -0.4662714048949997969 ) ) ;
#4685=CARTESIAN_POINT ( 'NONE',  ( 4.743586762672791224, -62.02470411057556277, -2.725691114197594800 ) ) ;
#4693=CARTESIAN_POINT ( 'NONE',  ( 5.216904734083789741, -62.90507476914316953, -1.366939949738901872 ) ) ;
#4694=CARTESIAN_POINT ( 'NONE',  ( 2.986904076224405014, -66.15109244657664078, 2.931604786918900363 ) ) ;
#4695=CARTESIAN_POINT ( 'NONE',  ( -14.07431766324681988, -37.03265636863024923, 1.026284428608169819 ) ) ;
#4702=CARTESIAN_POINT ( 'NONE',  ( -6.238986924797109701, -58.62463756020586914, -0.4569988612983747478 ) ) ;
#4714=CARTESIAN_POINT ( 'NONE',  ( 6.009612259771691889, -62.32653421013910133, 2.666676400654164336 ) ) ;
#4715=CARTESIAN_POINT ( 'NONE',  ( 4.394524616800664418, -62.98074765389134910, -0.6184872726264748488 ) ) ;
#4717=CARTESIAN_POINT ( 'NONE',  ( 3.771067679589467758, -56.05376814337366653, 0.3277224891452724109 ) ) ;
#4718=CARTESIAN_POINT ( 'NONE',  ( 3.533549941398215211, -54.99147314093924166, 0.1611374604154752754 ) ) ;
#4726=AXIS2_PLACEMENT_3D ( 'NONE', #4261, #3300, #5482 ) ;
#4727=CARTESIAN_POINT ( 'NONE',  ( 3.371673436877395069, -65.30458424753078361, -1.190358958913985798 ) ) ;
#4729=CARTESIAN_POINT ( 'NONE',  ( 3.660823140336725068, -65.74644859602665292, -1.309095517728299907 ) ) ;
#4730=CARTESIAN_POINT ( 'NONE',  ( 9.358334193258830425, -51.27205182843857045, -2.495037190209991707 ) ) ;
#4736=VECTOR ( 'NONE', #2425, 1000.000000000000114 ) ;
#4741=CARTESIAN_POINT ( 'NONE',  ( 3.942295684294244928, -66.34053734621645049, -3.017350621022677259 ) ) ;
#4742=CARTESIAN_POINT ( 'NONE',  ( 14.63724902514210058, -35.33341991383040437, 3.658178766884820465 ) ) ;
#4743=VECTOR ( 'NONE', #6740, 1000.000000000000000 ) ;
#4751=CARTESIAN_POINT ( 'NONE',  ( 1.700848490796859958, -66.65813550864595527, 0.8993149516912349872 ) ) ;
#4752=CARTESIAN_POINT ( 'NONE',  ( -4.423017985506799477, -63.40237279495851652, -1.015450938335749953 ) ) ;
#4755=CARTESIAN_POINT ( 'NONE',  ( -4.146345969758961303, -64.48517036809602132, -2.792927026443133620 ) ) ;
#4761=CARTESIAN_POINT ( 'NONE',  ( -1.592557218785495055, -66.68601476236933934, 1.076257986235874764 ) ) ;
#4762=CARTESIAN_POINT ( 'NONE',  ( -4.892892059336399591, -61.27075929137718191, 2.302341147961269652 ) ) ;
#4767=EDGE_CURVE ( 'NONE', #2618, #2328, #715, .T. ) ;
#4768=VERTEX_POINT ( 'NONE', #1178 ) ;
#4770=VERTEX_POINT ( 'NONE', #1808 ) ;
#4772=CARTESIAN_POINT ( 'NONE',  ( 6.643375263299909683, -62.64442119333418901, -2.502572238011808281 ) ) ;
#4774=CARTESIAN_POINT ( 'NONE',  ( 3.575547067216904740, -66.56692562923595347, -0.8973241761454349152 ) ) ;
#4776=ORIENTED_EDGE ( 'NONE', *, *, #5131, .F. ) ;
#4779=EDGE_LOOP ( 'NONE', ( #6574, #7367, #756, #4586, #5165, #570 ) ) ;
#4788=CARTESIAN_POINT ( 'NONE',  ( 4.514859508800350696, -57.62591736726079006, 0.04509635899271501047 ) ) ;
#4791=CARTESIAN_POINT ( 'NONE',  ( -3.433631738237976183, -65.10219846222973672, -0.7473139100181247496 ) ) ;
#4792=CARTESIAN_POINT ( 'NONE',  ( -6.272953878096410030, -61.45586155529391448, 1.493064301322690968 ) ) ;
#4797=DIRECTION ( 'NONE',  ( 0.9492883822130744331, -0.3144066910790611624, 0.000000000000000000 ) ) ;
#4799=CARTESIAN_POINT ( 'NONE',  ( -5.354034084503060065, -64.02545556441495478, -0.7792797212839647214 ) ) ;
#4807=AXIS2_PLACEMENT_3D ( 'NONE', #711, #2973, #3080 ) ;
#4809=CARTESIAN_POINT ( 'NONE',  ( -4.797760869400969241, -62.71499483963494015, 1.636667228454699696 ) ) ;
#4812=VERTEX_POINT ( 'NONE', #5251 ) ;
#4820=CARTESIAN_POINT ( 'NONE',  ( 5.361387189091391114, -62.18179348072126089, -1.559119044556545264 ) ) ;
#4821=CARTESIAN_POINT ( 'NONE',  ( -6.634274853075190492, -62.58082626503517787, -0.8104611758546799161 ) ) ;
#4825=CARTESIAN_POINT ( 'NONE',  ( -1.449391072403324099, -66.17791180637956927, 1.195139069250764852 ) ) ;
#4828=CARTESIAN_POINT ( 'NONE',  ( 3.369499982158394413, -65.21487972265850885, -3.264809282300078941 ) ) ;
#4836=CARTESIAN_POINT ( 'NONE',  ( 6.411082221499690093, -62.51743072077169217, -1.649542549651403789 ) ) ;
#4839=AXIS2_PLACEMENT_3D ( 'NONE', #492, #3947, #2214 ) ;
#4846=CARTESIAN_POINT ( 'NONE',  ( -2.818432829560444830, -65.09919931551695527, -0.6601304211325950133 ) ) ;
#4847=CARTESIAN_POINT ( 'NONE',  ( 5.838403032797286230, -57.93839583847110219, 2.430643543276013840 ) ) ;
#4852=VERTEX_POINT ( 'NONE', #645 ) ;
#4859=CARTESIAN_POINT ( 'NONE',  ( -6.752862897928530117, -62.17267392066884213, 1.309913053057485177 ) ) ;
#4867=CARTESIAN_POINT ( 'NONE',  ( -5.076816837522959425, -57.40733507789485657, 1.813788655352380541 ) ) ;
#4869=DIRECTION ( 'NONE',  ( 0.2223157560262044585, -0.6712493609847989262, 0.7071067811865449082 ) ) ;
#4871=CARTESIAN_POINT ( 'NONE',  ( 3.485917318579867974, -55.75437092160269259, -1.796392032914925441 ) ) ;
#4872=EDGE_CURVE ( 'NONE', #232, #2665, #4414, .T. ) ;
#4874=B_SPLINE_CURVE_WITH_KNOTS ( 'NONE', 3,
 ( #574, #1184, #1781, #5174, #6, #5860, #3466, #2297, #5779, #121, #6374, #1220, #3502, #653, #2941, #1813, #2974, #2408, #4717, #7005, #1849, #6002, #1912, #6476, #6514, #4299, #2563, #5318, #753, #2451, #3115, #6041, #5927, #5432, #5890, #1294, #4791, #195, #1881, #5971, #7111, #231, #267, #3004, #791, #7075, #1325, #7188, #4221, #6587, #5484, #820, #4871, #7153, #2599, #3655, #4265, #1396, #1364, #3048, #4907, #1990, #3081, #3610, #5394, #1426, #3717, #153, #5363, #4755, #861, #3159, #2487, #309, #712, #3576, #2523, #4828, #4185, #1949, #6557 ),
 .UNSPECIFIED., .F., .F.,
 ( 4, 2, 1, 2, 2, 2, 2, 2, 1, 2, 2, 2, 2, 2, 2, 1, 2, 2, 2, 2, 2, 2, 1, 2, 2, 2, 2, 1, 2, 2, 2, 2, 2, 2, 1, 2, 2, 2, 2, 2, 2, 1, 2, 4 ),
 ( 0.000000000000000000, 0.03124999999999918121, 0.06249999999999836242, 0.07812499999999794609, 0.09374999999999754363, 0.1249999999999967804, 0.1562499999999960032, 0.1874999999999954758, 0.2187499999999949207, 0.2343749999999947820, 0.2499999999999946154, 0.2812499999999942268, 0.2968749999999940603, 0.3124999999999938383, 0.3437499999999935052, 0.3749999999999931166, 0.3906249999999930611, 0.4062499999999929501, 0.4374999999999928391, 0.4531249999999930056, 0.4687499999999931721, 0.4999999999999934497, 0.5312499999999937828, 0.5468749999999937828, 0.5624999999999937828, 0.5937499999999940048, 0.6093749999999940048, 0.6249999999999940048, 0.6562499999999944489, 0.6874999999999948930, 0.7031249999999950040, 0.7187499999999951150, 0.7499999999999955591, 0.7656249999999956701, 0.7812499999999958922, 0.8124999999999960032, 0.8437499999999962252, 0.8593749999999965583, 0.8749999999999968914, 0.9062499999999977796, 0.9218749999999981126, 0.9374999999999985567, 0.9687499999999992228, 1.000000000000000000 ),
 .UNSPECIFIED. ) ;
#4880=CARTESIAN_POINT ( 'NONE',  ( -1.892846266465454841, -54.28526762408564110, -0.1610563749503846620 ) ) ;
#4881=CARTESIAN_POINT ( 'NONE',  ( 6.135463341229070444, -63.36916140199613778, -1.604994752452352014 ) ) ;
#4882=DIRECTION ( 'NONE',  ( -0.3144019573014847913, 0.9492899500389727629, 0.000000000000000000 ) ) ;
#4888=CARTESIAN_POINT ( 'NONE',  ( -4.780177894917470027, -57.84320307688069107, -2.250545046436859931 ) ) ;
#4890=CARTESIAN_POINT ( 'NONE',  ( 0.9559744929575736405, -54.27280436806401553, -0.007946376159375018178 ) ) ;
#4891=ORIENTED_EDGE ( 'NONE', *, *, #7247, .T. ) ;
#4896=DIRECTION ( 'NONE',  ( -0.9492899500389726519, -0.3144019573014848468, 0.000000000000000000 ) ) ;
#4899=CARTESIAN_POINT ( 'NONE',  ( -6.177752788274950113, -57.21669580536380550, -0.5454192084659099660 ) ) ;
#4901=DIRECTION ( 'NONE',  ( -0.3144066910790607183, -0.9492883822130744331, 0.000000000000000000 ) ) ;
#4902=CARTESIAN_POINT ( 'NONE',  ( 2.753836159791509974, -65.67748394244114252, 3.050484385245309849 ) ) ;
#4905=EDGE_CURVE ( 'NONE', #5349, #1972, #2198, .T. ) ;
#4907=CARTESIAN_POINT ( 'NONE',  ( -3.709322566982521607, -56.00042724521213700, -2.242165404915447358 ) ) ;
#4912=DIRECTION ( 'NONE',  ( 0.3144066910790611624, 0.9492883822130744331, 6.800116025829053242E-16 ) ) ;
#4913=DIRECTION ( 'NONE',  ( 0.9492899500389719858, 0.3144019573014870117, 0.000000000000000000 ) ) ;
#4914=CARTESIAN_POINT ( 'NONE',  ( -6.216708800954390490, -58.75440211775612909, 1.606470739968075545 ) ) ;
#4916=CARTESIAN_POINT ( 'NONE',  ( 1.530679711083600125, -53.64394877353957014, -0.1027361406249600040 ) ) ;
#4918=ORIENTED_EDGE ( 'NONE', *, *, #4872, .F. ) ;
#4921=CARTESIAN_POINT ( 'NONE',  ( -14.49899450467539985, -35.75040780681265318, -0.4662714048949997969 ) ) ;
#4924=CARTESIAN_POINT ( 'NONE',  ( -2.864422359069719981, -64.63427441546140528, 2.032225693688770374 ) ) ;
#4926=CARTESIAN_POINT ( 'NONE',  ( -4.691628851351036467, -64.57111108347837103, 3.374496055255405746 ) ) ;
#4934=CARTESIAN_POINT ( 'NONE',  ( -6.381106047699259598, -62.60757382768967716, 3.386766328596300113 ) ) ;
#4938=LINE ( 'NONE', #854, #151 ) ;
#4939=CARTESIAN_POINT ( 'NONE',  ( -6.216708800954390490, -58.75440211775612909, 1.606470739968075545 ) ) ;
#4941=DIRECTION ( 'NONE',  ( 0.3144019573014844582, -0.9492899500389728740, 0.000000000000000000 ) ) ;
#4944=VERTEX_POINT ( 'NONE', #5031 ) ;
#4949=CARTESIAN_POINT ( 'NONE',  ( -5.799935258789999715, -64.30794688765904255, -0.8981536636440297094 ) ) ;
#4950=DIRECTION ( 'NONE',  ( 0.9492883822130744331, -0.3144066910790611624, 0.000000000000000000 ) ) ;
#4957=CARTESIAN_POINT ( 'NONE',  ( -5.172139827190740391, -61.55016382346040871, 1.714186298074440007 ) ) ;
#4959=CARTESIAN_POINT ( 'NONE',  ( -5.129009619570435774, -56.77828967133876858, 1.722487601996475881 ) ) ;
#4960=CARTESIAN_POINT ( 'NONE',  ( 5.944105978113960020, -62.47685828501489169, -3.593838583070729786 ) ) ;
#4969=CARTESIAN_POINT ( 'NONE',  ( -6.708998324124310741, -61.63987295270813860, 3.437611327301279385 ) ) ;
#4983=CIRCLE ( 'NONE', #5958, 1.000000000000000444 ) ;
#4984=DIRECTION ( 'NONE',  ( 0.2223191033124284066, 0.6712482523644728305, 0.7071067811865466846 ) ) ;
#4985=EDGE_CURVE ( 'NONE', #380, #1089, #6496, .T. ) ;
#4987=AXIS2_PLACEMENT_3D ( 'NONE', #39, #3642, #739 ) ;
#4989=CARTESIAN_POINT ( 'NONE',  ( -7.067610632470020526, -58.47094543896879060, 0.9162228916581999227 ) ) ;
#4994=LINE ( 'NONE', #5604, #7120 ) ;
#4996=EDGE_CURVE ( 'NONE', #327, #3172, #4338, .T. ) ;
#4997=CARTESIAN_POINT ( 'NONE',  ( 2.303277369485650095, -64.96541665026637702, 1.677260903589945285 ) ) ;
#5008=CARTESIAN_POINT ( 'NONE',  ( 6.378760423371060639, -64.06988568591069111, -0.05691440262071967293 ) ) ;
#5013=CARTESIAN_POINT ( 'NONE',  ( 1.316624512147740012, -66.75104842734066324, 3.019790780136459851 ) ) ;
#5016=ORIENTED_EDGE ( 'NONE', *, *, #6874, .T. ) ;
#5021=CARTESIAN_POINT ( 'NONE',  ( -3.941959611298590183, -54.25574829393653431, -0.9393447306324897994 ) ) ;
#5026=CARTESIAN_POINT ( 'NONE',  ( -4.954937549494499827, -61.85628170826059602, 3.287035460711430268 ) ) ;
#5029=CARTESIAN_POINT ( 'NONE',  ( -5.038070929474960380, -61.61169989543196834, 3.303768584289609844 ) ) ;
#5031=CARTESIAN_POINT ( 'NONE',  ( 14.81352433457121975, -34.80119172639020064, 2.597518595105000383 ) ) ;
#5041=CARTESIAN_POINT ( 'NONE',  ( -6.841972559203830961, -62.34857902771452842, 2.832214187714990228 ) ) ;
#5043=EDGE_CURVE ( 'NONE', #3646, #5842, #6618, .T. ) ;
#5045=EDGE_CURVE ( 'NONE', #1906, #5376, #500, .T. ) ;
#5046=CARTESIAN_POINT ( 'NONE',  ( 14.85956812845453889, -34.66217166146590500, 2.951071985698260125 ) ) ;
#5047=CARTESIAN_POINT ( 'NONE',  ( 5.447354608442940282, -62.18425133612383604, -1.411124226719259855 ) ) ;
#5050=CARTESIAN_POINT ( 'NONE',  ( -5.480856739662490540, -62.25220485324549458, 1.560007870815685260 ) ) ;
#5051=ORIENTED_EDGE ( 'NONE', *, *, #440, .F. ) ;
#5052=B_SPLINE_CURVE_WITH_KNOTS ( 'NONE', 3,
 ( #1897, #6495, #948, #7269, #915, #6464 ),
 .UNSPECIFIED., .F., .F.,
 ( 4, 2, 4 ),
 ( 0.000000000000000000, 0.5000000000000016653, 1.000000000000000000 ),
 .UNSPECIFIED. ) ;
#5057=CARTESIAN_POINT ( 'NONE',  ( -15.08175531864075047, -33.99084820126180517, -5.041145139047909396 ) ) ;
#5059=CIRCLE ( 'NONE', #3369, 0.9999999999999984457 ) ;
#5060=CARTESIAN_POINT ( 'NONE',  ( 6.251545776960879763, -56.60079747432034480, -0.4089935619396500299 ) ) ;
#5064=CARTESIAN_POINT ( 'NONE',  ( -4.930053471857299918, -61.64676491032937378, 0.1765652348176402209 ) ) ;
#5065=AXIS2_PLACEMENT_3D ( 'NONE', #4695, #4665, #1791 ) ;
#5068=CARTESIAN_POINT ( 'NONE',  ( -1.128062821581302000, -55.49617455686423284, 0.7066123397475153611 ) ) ;
#5071=ORIENTED_EDGE ( 'NONE', *, *, #6598, .T. ) ;
#5072=ORIENTED_EDGE ( 'NONE', *, *, #5701, .F. ) ;
#5074=DIRECTION ( 'NONE',  ( 0.9492883822130744331, -0.3144066910790611624, 0.000000000000000000 ) ) ;
#5075=AXIS2_PLACEMENT_3D ( 'NONE', #1555, #2719, #7345 ) ;
#5079=CARTESIAN_POINT ( 'NONE',  ( -3.328771606340945155, -66.98264282425255089, -1.647280098378362867 ) ) ;
#5080=ADVANCED_FACE ( 'NONE', ( #4122 ), #4628, .T. ) ;
#5082=AXIS2_PLACEMENT_3D ( 'NONE', #946, #272, #4269 ) ;
#5083=CIRCLE ( 'NONE', #1829, 1.000000000000000000 ) ;
#5091=ADVANCED_FACE ( 'NONE', ( #18 ), #3478, .T. ) ;
#5092=CARTESIAN_POINT ( 'NONE',  ( -5.895255198864449930, -62.39547700480248693, 1.556969243713622220 ) ) ;
#5093=MECHANICAL_DESIGN_GEOMETRIC_PRESENTATION_REPRESENTATION('',(#6412),#5942);
#5094=ORIENTED_EDGE ( 'NONE', *, *, #7245, .F. ) ;
#5096=TOROIDAL_SURFACE ( 'NONE', #2560, 1.500000000000000000, 1.000000000000000000 ) ;
#5100=AXIS2_PLACEMENT_3D ( 'NONE', #6826, #3966, #7348 ) ;
#5103=CARTESIAN_POINT ( 'NONE',  ( -6.891320273265630014, -62.11321098440852495, -0.2797727661029551505 ) ) ;
#5109=CARTESIAN_POINT ( 'NONE',  ( -1.630661209647960019, -65.50972637651682362, 2.960670344429949807 ) ) ;
#5113=FACE_OUTER_BOUND ( 'NONE', #1538, .T. ) ;
#5114=CARTESIAN_POINT ( 'NONE',  ( 4.394524616800664418, -62.98074765389134910, -0.6184872726264748488 ) ) ;
#5119=AXIS2_PLACEMENT_3D ( 'NONE', #2512, #3220, #1978 ) ;
#5125=CARTESIAN_POINT ( 'NONE',  ( 14.49911764349215915, -35.75048010860329839, 0.4975185951050001831 ) ) ;
#5127=CARTESIAN_POINT ( 'NONE',  ( 1.455885123031280148, -67.63619251397972221, 2.328451870335179752 ) ) ;
#5130=DIRECTION ( 'NONE',  ( 0.3144066910790611624, 0.9492883822130744331, 0.000000000000000000 ) ) ;
#5131=EDGE_CURVE ( 'NONE', #5892, #6872, #1221, .T. ) ;
#5132=CARTESIAN_POINT ( 'NONE',  ( 9.311407240687648468, -51.41373841511900622, -2.502481404895003259 ) ) ;
#5142=CARTESIAN_POINT ( 'NONE',  ( 14.63724902514211834, -35.33341991383040437, 3.658178766884810251 ) ) ;
#5143=CARTESIAN_POINT ( 'NONE',  ( -6.126235009943979293, -64.48141016635396738, -1.469515951087519978 ) ) ;
#5151=CARTESIAN_POINT ( 'NONE',  ( 4.230506805399654624, -63.24565307424497007, 1.502053860026275167 ) ) ;
#5153=CARTESIAN_POINT ( 'NONE',  ( 5.927764221498110331, -62.35749858221746678, -1.529935281190306862 ) ) ;
#5164=CARTESIAN_POINT ( 'NONE',  ( 3.751014749966880224, -66.74975575182239140, 0.1208598729073953049 ) ) ;
#5165=ORIENTED_EDGE ( 'NONE', *, *, #4549, .F. ) ;
#5174=CARTESIAN_POINT ( 'NONE',  ( -3.435267632410309080, -65.16561242980966995, 1.350366576929741491 ) ) ;
#5175=CARTESIAN_POINT ( 'NONE',  ( -4.011890603535904987, -66.29221981733677183, 1.575336318554399595 ) ) ;
#5179=ORIENTED_EDGE ( 'NONE', *, *, #1043, .F. ) ;
#5185=CARTESIAN_POINT ( 'NONE',  ( -4.773669824303439668, -63.68048849998092464, 3.536592896228280214 ) ) ;
#5195=CARTESIAN_POINT ( 'NONE',  ( 3.189415849367489564, -54.78201482374456788, -1.959602550130806753 ) ) ;
#5197=CARTESIAN_POINT ( 'NONE',  ( 1.340549191775572080, -65.71857943717337491, -0.9252791854465649557 ) ) ;
#5206=DIRECTION ( 'NONE',  ( -0.2163384215910431896, -0.07165063022625259292, 0.9736857165079894072 ) ) ;
#5222=EDGE_CURVE ( 'NONE', #5376, #1906, #1100, .T. ) ;
#5226=CARTESIAN_POINT ( 'NONE',  ( -3.268634523084565036, -65.37612200555487618, 3.404282007464019877 ) ) ;
#5228=AXIS2_PLACEMENT_3D ( 'NONE', #5125, #1049, #3301 ) ;
#5229=CARTESIAN_POINT ( 'NONE',  ( -5.206993624623629913, -63.95781028998001716, 3.417603084305509853 ) ) ;
#5239=CARTESIAN_POINT ( 'NONE',  ( -3.365275581743949918, -66.00192919971716776, -0.8990674732841750227 ) ) ;
#5241=CARTESIAN_POINT ( 'NONE',  ( 5.253257825778660184, -59.02147093648149223, -1.455491405082765866 ) ) ;
#5251=CARTESIAN_POINT ( 'NONE',  ( -15.49899450467540163, -35.75040780681265318, -0.4662714048949997969 ) ) ;
#5252=EDGE_CURVE ( 'NONE', #5988, #6077, #3011, .T. ) ;
#5253=CARTESIAN_POINT ( 'NONE',  ( -1.005393588828258133, -65.41824993351924888, -2.298700180912566449 ) ) ;
#5256=B_SPLINE_SURFACE_WITH_KNOTS ( 'NONE', 3, 3, ( 
 ( #2371, #783, #3569, #5357, #6504, #1876, #189, #4214, #3073, #5884, #5310, #4678, #1350, #6369, #1213, #6962, #705, #4102, #5856, #3494, #2995, #644, #2935, #6405, #4751, #3540, #7258, #7144, #3821, #6112, #6076, #4324, #2551, #3677, #6658, #224, #3105, #7100, #3186, #934, #1456, #7180, #898, #2664, #1505 ),
 ( #4969, #3790, #969, #4934, #5995, #2099, #1421, #1936, #4407, #4252, #3146, #5512, #1980, #6033, #5425, #335, #6695, #6580, #258, #1536, #4859, #6548, #2052, #3711, #4291, #850, #2514, #5470, #300, #4366, #6143, #2015, #5389, #2592, #4899, #6615, #4821, #1390, #3748, #2625, #7218, #3222, #5542, #371, #5577 ),
 ( #525, #2846, #5041, #2706, #6288, #1051, #1128, #2810, #5127, #6219, #3303, #3339, #2126, #7325, #5688, #5651, #2166, #6882, #4557, #7405, #1728, #4477, #414, #4027, #3418, #5164, #5008, #6763, #6252, #6179, #486, #2284, #1615, #1088, #2766, #7290, #4438, #1013, #5079, #4525, #2250, #1573, #7364, #3905, #5620 ),
 ( #5734, #4597, #6841, #1685, #3982, #6328, #2210, #3375, #454, #7440, #3258, #3860, #2734, #6806, #1648, #3942, #562, #1240, #6327, #135, #5301, #2959, #5848, #732, #630, #4774, #7030, #6988, #5272, #3484, #4638, #2429, #1167, #1764, #591, #4133, #1868, #2392, #672, #1831, #3593, #4741, #1896, #4172, #2325 ),
 ( #29, #6434, #1282, #4091, #5907, #2362, #5802, #1202, #5763, #102, #4059, #3451, #6360, #6925, #2920, #3560, #3525, #5875, #2472, #4702, #699, #2988, #5239, #6463, #1308, #3025, #2879, #5344, #7064, #179, #5195, #71, #4671, #6953, #1797, #6396, #6643, #246, #3630, #1412, #3211, #6537, #777, #4202, #3701 ),
 ( #5952, #4957, #1490, #2539, #4809, #5383, #3175, #215, #7091, #807, #6020, #2042, #1444, #885, #2650, #3132, #2615, #1382, #5500, #6604, #359, #324, #4846, #6494, #1342, #6100, #7134, #3670, #838, #4238, #3778, #2006, #2505, #1926, #4888, #3066, #5987, #5452, #1969, #3096, #289, #7169, #5412, #923, #5531 ),
 ( #4315, #6060, #4281, #7243, #6572, #2582, #4924, #7206, #4351, #4997, #5151, #7277, #3248, #5565, #4511, #6751, #5068, #5720, #1038, #6793, #3893, #2116, #3326, #3363, #473, #1525, #5114, #550, #7394, #2195, #6132, #441, #2753, #3811, #400, #4545, #5605, #957, #1605, #1113, #4427, #2693, #2088, #6207, #7312 ),
 ( #1637, #5029, #6167, #2834, #5675, #3927, #4395, #996, #6683, #6715, #2238, #3967, #1559, #2724, #7350, #3848, #2152, #3403, #3289, #513, #4464, #5640, #2796, #6827, #1671, #6277, #4120, #4010, #6947, #5790, #16, #723, #3583, #1270, #6978, #5897, #4051, #2270, #3014, #2979, #1859, #6866, #3476, #2948, #2868 ),
 ( #1193, #5263, #2907, #1711, #6317, #5185, #5226, #1228, #6423, #1158, #1789, #617, #2309, #7428, #62, #5293, #6453, #1821, #3550, #5866, #4581, #4663, #94, #4625, #4162, #1298, #3441, #6915, #6384, #1755, #2354, #127, #4081, #5753, #690, #2418, #3513, #5834, #583, #6351, #662, #4727, #2383, #4693, #7017 ),
 ( #167, #764, #7052, #3123, #870, #1403, #7122, #828, #2606, #1433, #914, #4306, #1333, #798, #6009, #6483, #5440, #276, #3087, #4914, #1371, #2494, #203, #4761, #4273, #3057, #5329, #5371, #3618, #5936, #2573, #2530, #4880, #1476, #6563, #7159, #1959, #4799, #3690, #6594, #1998, #1887, #3166, #3767, #5492 ) ),
 .UNSPECIFIED., .T., .F., .F.,
 ( 4, 2, 2, 2, 4 ),
 ( 4, 3, 2, 2, 2, 2, 2, 2, 2, 2, 2, 2, 2, 2, 2, 2, 2, 2, 2, 2, 2, 4 ),
 ( 0.000000000000000000, 0.2500000000000000000, 0.5000000000000000000, 0.7500000000000000000, 1.000000000000000000 ),
 ( -0.01000000000000000021, 0.000000000000000000, 0.02628634692406570106, 0.07896140836526269191, 0.1315838524972270107, 0.1842089079736879964, 0.2368304666025229932, 0.2894621644501310098, 0.3421084969797454911, 0.3947501728568885149, 0.4473769119526340154, 0.5000000000000000000, 0.5526230880473660401, 0.6052498271431119292, 0.6578915030202550085, 0.7105378355498690457, 0.7631695333974770623, 0.8157910920263119481, 0.8684161475027730726, 0.9210385916347370028, 0.9737136530759340491, 1.000000000000000000 ),
 .UNSPECIFIED. ) ;
#5257=CARTESIAN_POINT ( 'NONE',  ( -6.321361399357500410, -61.94876894069515316, -0.6341497168666246909 ) ) ;
#5260=CARTESIAN_POINT ( 'NONE',  ( -5.904042796847299712, -62.42803713013675093, 3.506543003539000392 ) ) ;
#5263=CARTESIAN_POINT ( 'NONE',  ( -5.595710845088040841, -61.75488600311453524, 3.658668618637090031 ) ) ;
#5264=CARTESIAN_POINT ( 'NONE',  ( -1.206827191127304078, -66.77204028133226643, -1.044217440639481742 ) ) ;
#5269=VERTEX_POINT ( 'NONE', #2033 ) ;
#5272=CARTESIAN_POINT ( 'NONE',  ( 6.836834775951150078, -58.56388191083841122, -1.340052733437185895 ) ) ;
#5276=( LENGTH_UNIT ( ) NAMED_UNIT ( * ) SI_UNIT ( .MILLI., .METRE. ) );
#5281=CARTESIAN_POINT ( 'NONE',  ( -9.311346830843410416, -51.41373841511902043, 2.533728595105000370 ) ) ;
#5282=ORIENTED_EDGE ( 'NONE', *, *, #738, .T. ) ;
#5285=CARTESIAN_POINT ( 'NONE',  ( 1.159677199572074269, -55.50330010691895666, -1.238196965061255650 ) ) ;
#5287=CARTESIAN_POINT ( 'NONE',  ( 5.463696144088109996, -62.30361170774578028, -3.475027489484119769 ) ) ;
#5293=CARTESIAN_POINT ( 'NONE',  ( 1.626596344682255113, -54.75750786503496670, 2.255510009909589719 ) ) ;
#5294=CARTESIAN_POINT ( 'NONE',  ( -5.354034084503060065, -64.02545556441495478, -0.7792797212839647214 ) ) ;
#5297=ORIENTED_EDGE ( 'NONE', *, *, #3679, .T. ) ;
#5299=DIRECTION ( 'NONE',  ( 0.3128463504745289114, 0.9445772445362836667, 0.09950371902099885979 ) ) ;
#5301=CARTESIAN_POINT ( 'NONE',  ( -6.891320273265630014, -62.11321098440852495, -0.2797727661029551505 ) ) ;
#5307=ADVANCED_FACE ( 'NONE', ( #4308 ), #3169, .T. ) ;
#5309=CARTESIAN_POINT ( 'NONE',  ( 5.930474762900869834, -62.46354786334135412, -3.475732462342234985 ) ) ;
#5310=CARTESIAN_POINT ( 'NONE',  ( 5.416018991692120643, -63.93240027730202968, 2.754852738177090643 ) ) ;
#5311=EDGE_LOOP ( 'NONE', ( #5535, #4018, #4567, #7237, #906, #5796 ) ) ;
#5313=CARTESIAN_POINT ( 'NONE',  ( 2.751515497641074948, -64.99867735210931130, 0.5749532485596650089 ) ) ;
#5318=CARTESIAN_POINT ( 'NONE',  ( -4.705238872764143210, -56.98302411029121828, -0.2229714063405454361 ) ) ;
#5319=CARTESIAN_POINT ( 'NONE',  ( -5.727966693761760375, -63.15494832584334262, 1.398024598501910187 ) ) ;
#5323=DIRECTION ( 'NONE',  ( -0.3144019573014841806, 0.9492899500389728740, 0.000000000000000000 ) ) ;
#5324=EDGE_CURVE ( 'NONE', #2342, #5842, #5803, .T. ) ;
#5329=CARTESIAN_POINT ( 'NONE',  ( 5.619938529503549773, -63.59344562873818774, 0.6343307546824898946 ) ) ;
#5331=CARTESIAN_POINT ( 'NONE',  ( 3.331090576803830139, -65.95739139720836874, 0.8111086825117052035 ) ) ;
#5336=ORIENTED_EDGE ( 'NONE', *, *, #6230, .T. ) ;
#5340=LINE ( 'NONE', #7089, #994 ) ;
#5344=CARTESIAN_POINT ( 'NONE',  ( 6.291895255447879975, -62.07086823355334104, -1.517278733858541839 ) ) ;
#5349=VERTEX_POINT ( 'NONE', #6094 ) ;
#5353=DIRECTION ( 'NONE',  ( -0.3144019573014843472, 0.9492899500389728740, 0.000000000000000000 ) ) ;
#5357=CARTESIAN_POINT ( 'NONE',  ( -5.895051854024569771, -62.45358532148892294, 3.505907163650189950 ) ) ;
#5360=CARTESIAN_POINT ( 'NONE',  ( -2.961840227416660198, -65.56364223063081909, 1.283932781279834900 ) ) ;
#5362=CARTESIAN_POINT ( 'NONE',  ( 4.814269575835951720, -62.05762139399459443, -2.948265134628040407 ) ) ;
#5363=CARTESIAN_POINT ( 'NONE',  ( -4.722210582817570668, -63.78749880788215876, -2.740498917967187698 ) ) ;
#5364=CARTESIAN_POINT ( 'NONE',  ( 1.600318488538475137, -66.74162401608067796, -1.164216807110747931 ) ) ;
#5371=CARTESIAN_POINT ( 'NONE',  ( 6.265638173095489982, -61.94185186372677521, 0.5461908750427398873 ) ) ;
#5372=CARTESIAN_POINT ( 'NONE',  ( -4.747117373927349782, -63.10583374278928659, -0.4844647803776696016 ) ) ;
#5373=CARTESIAN_POINT ( 'NONE',  ( -5.895051854024569771, -62.45358532148892294, 3.505907163650189950 ) ) ;
#5376=VERTEX_POINT ( 'NONE', #2745 ) ;
#5383=CARTESIAN_POINT ( 'NONE',  ( -4.450126406946254498, -63.33667035482537244, 1.592103300391294773 ) ) ;
#5388=CARTESIAN_POINT ( 'NONE',  ( 5.001731546698911401, -62.07693240093809806, -1.811760589978133051 ) ) ;
#5389=CARTESIAN_POINT ( 'NONE',  ( -2.038541806680159940, -53.77797276486428046, -0.2805255711276150588 ) ) ;
#5391=CARTESIAN_POINT ( 'NONE',  ( -1.397697773942189858, -54.69607029038206747, 2.078897745975250455 ) ) ;
#5394=CARTESIAN_POINT ( 'NONE',  ( -5.758700247327861454, -59.47069914579707017, -2.478271157609042596 ) ) ;
#5402=CARTESIAN_POINT ( 'NONE',  ( 3.949972843796054178, -66.18831294452250802, -1.427832076542613793 ) ) ;
#5405=VERTEX_POINT ( 'NONE', #545 ) ;
#5406=ORIENTED_EDGE ( 'NONE', *, *, #5689, .T. ) ;
#5412=CARTESIAN_POINT ( 'NONE',  ( 4.396896920912054973, -63.41639021975223045, -3.266830536337445245 ) ) ;
#5413=CARTESIAN_POINT ( 'NONE',  ( 3.692193437564742275, -55.33181466697134709, 0.1491418217178651084 ) ) ;
#5415=ORIENTED_EDGE ( 'NONE', *, *, #5131, .T. ) ;
#5417=ORIENTED_EDGE ( 'NONE', *, *, #303, .T. ) ;
#5421=EDGE_CURVE ( 'NONE', #6025, #5269, #2567, .T. ) ;
#5425=CARTESIAN_POINT ( 'NONE',  ( 3.691078954254495059, -54.53160935192415337, 2.105200478230089267 ) ) ;
#5427=AXIS2_PLACEMENT_3D ( 'NONE', #3516, #5755, #5792 ) ;
#5429=CARTESIAN_POINT ( 'NONE',  ( -4.559578989909869762, -57.69789612496867903, 1.459412177499654462 ) ) ;
#5432=CARTESIAN_POINT ( 'NONE',  ( -5.212048506017270100, -63.07061735744050424, -0.5901561396984810193 ) ) ;
#5440=CARTESIAN_POINT ( 'NONE',  ( -1.512046953658800152, -54.18079592905042574, 1.959428465566195543 ) ) ;
#5441=CARTESIAN_POINT ( 'NONE',  ( -3.403807323753265113, -54.36107883567960641, 1.752763223655470437 ) ) ;
#5446=ORIENTED_EDGE ( 'NONE', *, *, #3053, .F. ) ;
#5452=CARTESIAN_POINT ( 'NONE',  ( -4.574768583212910578, -63.39215034952142247, -2.605000795493774834 ) ) ;
#5453=CARTESIAN_POINT ( 'NONE',  ( 3.293998498883576875, -65.74688398529977462, 0.8048007446836616952 ) ) ;
#5457=ORIENTED_EDGE ( 'NONE', *, *, #5607, .T. ) ;
#5466=CIRCLE ( 'NONE', #2329, 1.000000000000000000 ) ;
#5469=CARTESIAN_POINT ( 'NONE',  ( 4.748085323256989732, -62.01668842780453872, -2.502390571778199568 ) ) ;
#5470=CARTESIAN_POINT ( 'NONE',  ( 6.775879105374429834, -62.07729961717699041, 0.4273099905340951299 ) ) ;
#5474=ORIENTED_EDGE ( 'NONE', *, *, #2873, .T. ) ;
#5479=CARTESIAN_POINT ( 'NONE',  ( -5.250750166908019878, -57.72135505925717069, -0.3064819419056146188 ) ) ;
#5482=DIRECTION ( 'NONE',  ( 1.000000000000000000, 0.000000000000000000, 0.000000000000000000 ) ) ;
#5483=CARTESIAN_POINT ( 'NONE',  ( 14.49911764349215915, -35.75048010860329839, 2.597518595105000383 ) ) ;
#5484=CARTESIAN_POINT ( 'NONE',  ( 5.463205525817310892, -58.24907413091714403, -1.612795058816904437 ) ) ;
#5490=CARTESIAN_POINT ( 'NONE',  ( -14.07431766324681988, -37.03265636863024923, 1.026284428608169819 ) ) ;
#5492=CARTESIAN_POINT ( 'NONE',  ( 5.929218414971320072, -62.35084102844776055, -1.530333388185332932 ) ) ;
#5494=CARTESIAN_POINT ( 'NONE',  ( 3.357456528971034970, -66.96770758659590683, 2.241359037429140333 ) ) ;
#5500=CARTESIAN_POINT ( 'NONE',  ( -4.614416121558960526, -57.55752852796073427, -0.1302737383155048445 ) ) ;
#5503=CARTESIAN_POINT ( 'NONE',  ( -0.06384554175070766835, -54.19636094766362078, 2.037209790278620591 ) ) ;
#5510=B_SPLINE_CURVE_WITH_KNOTS ( 'NONE', 3,
 ( #3832, #3349, #5589, #1467, #5627, #459, #426, #2712, #5092, #944, #3760, #5050 ),
 .UNSPECIFIED., .F., .F.,
 ( 4, 2, 2, 2, 2, 4 ),
 ( 0.000000000000000000, 0.1249999999999981404, 0.2499999999999962808, 0.4999999999999954481, 0.7499999999999976685, 1.000000000000000000 ),
 .UNSPECIFIED. ) ;
#5512=CARTESIAN_POINT ( 'NONE',  ( 6.663059173928499668, -62.48704134639812935, 2.547684199221960100 ) ) ;
#5515=CARTESIAN_POINT ( 'NONE',  ( 5.661113010068490325, -57.37064013373739613, 2.401523511004880262 ) ) ;
#5522=FACE_OUTER_BOUND ( 'NONE', #4309, .T. ) ;
#5525=CARTESIAN_POINT ( 'NONE',  ( 6.802585521241110378, -58.92636561181245014, 2.370308086683080351 ) ) ;
#5529=DIRECTION ( 'NONE',  ( -0.5224671166576538850, 0.8526594349512809368, 0.000000000000000000 ) ) ;
#5531=CARTESIAN_POINT ( 'NONE',  ( 4.980378365057210210, -62.14367890036703557, -3.355420260138584521 ) ) ;
#5533=CARTESIAN_POINT ( 'NONE',  ( -5.001340985743557788, -64.18787007827532420, 3.400789707794877881 ) ) ;
#5534=CARTESIAN_POINT ( 'NONE',  ( -1.334494426138621792, -66.80443255658586565, -3.107681693547102775 ) ) ;
#5535=ORIENTED_EDGE ( 'NONE', *, *, #217, .F. ) ;
#5542=CARTESIAN_POINT ( 'NONE',  ( 5.693513582185560473, -64.15546253253084785, -1.561391656022143914 ) ) ;
#5547=CARTESIAN_POINT ( 'NONE',  ( 1.700848490796859958, -66.65813550864595527, 0.8993149516912349872 ) ) ;
#5551=AXIS2_PLACEMENT_3D ( 'NONE', #692, #129, #1890 ) ;
#5552=ORIENTED_EDGE ( 'NONE', *, *, #2131, .F. ) ;
#5558=CARTESIAN_POINT ( 'NONE',  ( -6.268616217933410617, -56.62827303305337523, 1.003072567477500066 ) ) ;
#5565=CARTESIAN_POINT ( 'NONE',  ( 4.485945982887084682, -58.07227379738043993, 1.147183751133595386 ) ) ;
#5577=CARTESIAN_POINT ( 'NONE',  ( 6.411082221499690093, -62.51743072077169217, -1.649542549651403789 ) ) ;
#5584=CARTESIAN_POINT ( 'NONE',  ( -3.498019654714389581, -55.03494779767484602, -0.2490962732230048438 ) ) ;
#5589=CARTESIAN_POINT ( 'NONE',  ( -6.630541856184143157, -62.63987563302658401, 2.331428407641557676 ) ) ;
#5592=ADVANCED_BREP_SHAPE_REPRESENTATION ( '', ( #7333, #751 ), #6896 ) ;
#5597=DIRECTION ( 'NONE',  ( 0.3144019573014849023, -0.9492899500389726519, 0.000000000000000000 ) ) ;
#5598=CARTESIAN_POINT ( 'NONE',  ( 6.071255580768259108, -56.77894568653594121, -1.427178034550365959 ) ) ;
#5604=CARTESIAN_POINT ( 'NONE',  ( -15.08175531864075047, -34.71610473016205134, -5.729623873133089518 ) ) ;
#5605=CARTESIAN_POINT ( 'NONE',  ( -4.847093383240289377, -61.94486680083809205, -1.943810276119404046 ) ) ;
#5607=EDGE_CURVE ( 'NONE', #1033, #7272, #1954, .T. ) ;
#5610=CARTESIAN_POINT ( 'NONE',  ( -5.010373352768399791, -62.05347898811812968, 1.680690861613699516 ) ) ;
#5616=ORIENTED_EDGE ( 'NONE', *, *, #3425, .F. ) ;
#5620=CARTESIAN_POINT ( 'NONE',  ( 6.738276468386390050, -62.65933952543014129, -2.221138621355481568 ) ) ;
#5622=CARTESIAN_POINT ( 'NONE',  ( -14.63712380658832046, -35.33334692323139592, -3.626931576674818025 ) ) ;
#5626=DIRECTION ( 'NONE',  ( 0.3128463504745289114, 0.9445772445362836667, 0.09950371902099885979 ) ) ;
#5627=CARTESIAN_POINT ( 'NONE',  ( -6.535529569156460106, -62.60774289024404027, 2.066694991760122502 ) ) ;
#5632=CARTESIAN_POINT ( 'NONE',  ( -5.788105944719140084, -64.22553544194731501, 1.709038299673605321 ) ) ;
#5636=CARTESIAN_POINT ( 'NONE',  ( 2.303277369485650095, -64.96541665026637702, 1.677260903589945285 ) ) ;
#5640=CARTESIAN_POINT ( 'NONE',  ( -4.596296085628660322, -63.12536419624139938, 1.105086706205665070 ) ) ;
#5644=ORIENTED_EDGE ( 'NONE', *, *, #5701, .T. ) ;
#5647=ADVANCED_FACE ( 'NONE', ( #1815 ), #5824, .T. ) ;
#5651=CARTESIAN_POINT ( 'NONE',  ( 2.082020516433249924, -53.40759131075155608, 1.446381639928540297 ) ) ;
#5653=FACE_OUTER_BOUND ( 'NONE', #482, .T. ) ;
#5655=CARTESIAN_POINT ( 'NONE',  ( -5.794328821513979655, -59.26142744441108334, -0.3953236866292048068 ) ) ;
#5663=CYLINDRICAL_SURFACE ( 'NONE', #5930, 0.9999999999999988898 ) ;
#5667=CARTESIAN_POINT ( 'NONE',  ( -6.519675230953620115, -62.56018929471859735, 1.797154853076760261 ) ) ;
#5671=CARTESIAN_POINT ( 'NONE',  ( 4.230506805399654624, -63.24565307424497007, 1.502053860026275167 ) ) ;
#5673=CARTESIAN_POINT ( 'NONE',  ( 15.08188723176695056, -34.71618050577090031, 5.760870465243799643 ) ) ;
#5675=CARTESIAN_POINT ( 'NONE',  ( -4.653276882800380321, -62.74377975942224595, 3.226317067983300202 ) ) ;
#5677=CARTESIAN_POINT ( 'NONE',  ( 2.420475147787775505, -66.32055832903793657, -1.240572518232158972 ) ) ;
#5688=CARTESIAN_POINT ( 'NONE',  ( 3.914764119449064772, -54.23824460091720567, 1.533423736523834346 ) ) ;
#5689=EDGE_CURVE ( 'NONE', #123, #5269, #7259, .T. ) ;
#5700=CIRCLE ( 'NONE', #1597, 1.000000000000000444 ) ;
#5701=EDGE_CURVE ( 'NONE', #6909, #2342, #1372, .T. ) ;
#5708=DIRECTION ( 'NONE',  ( 0.000000000000000000, -0.7252565289002705917, -0.6884787340851793447 ) ) ;
#5710=CARTESIAN_POINT ( 'NONE',  ( -3.268733238405740149, -66.73531384189965365, -2.665188268689791862 ) ) ;
#5714=VECTOR ( 'NONE', #1241, 999.9999999999998863 ) ;
#5719=CARTESIAN_POINT ( 'NONE',  ( -13.49899450467539985, -35.75040780681265318, -2.566271404894997499 ) ) ;
#5720=CARTESIAN_POINT ( 'NONE',  ( -2.437747074861595031, -55.99259917890189797, 0.6173017669495700632 ) ) ;
#5723=ORIENTED_EDGE ( 'NONE', *, *, #5222, .T. ) ;
#5724=ORIENTED_EDGE ( 'NONE', *, *, #1767, .T. ) ;
#5734=CARTESIAN_POINT ( 'NONE',  ( -6.840816475388580287, -61.57127885238590892, 1.848044054229609934 ) ) ;
#5745=DIRECTION ( 'NONE',  ( 0.2223191033124283789, 0.6712482523644727195, 0.7071067811865466846 ) ) ;
#5746=CARTESIAN_POINT ( 'NONE',  ( -6.921793923077749433, -58.90709844370859116, -2.222636374480685184 ) ) ;
#5748=ORIENTED_EDGE ( 'NONE', *, *, #7190, .F. ) ;
#5753=CARTESIAN_POINT ( 'NONE',  ( -3.222464925939095171, -55.48519077065235194, -0.1302151132178846482 ) ) ;
#5755=DIRECTION ( 'NONE',  ( 2.857391495672265093E-16, 4.793132013414519254E-17, 1.000000000000000000 ) ) ;
#5756=ORIENTED_EDGE ( 'NONE', *, *, #3822, .T. ) ;
#5763=CARTESIAN_POINT ( 'NONE',  ( 1.211170193666210038, -66.82801115824167937, 0.9562527914032201704 ) ) ;
#5765=CARTESIAN_POINT ( 'NONE',  ( -2.876828494605734754, -55.82398600891924190, -2.074803592940099861 ) ) ;
#5771=CARTESIAN_POINT ( 'NONE',  ( 15.49911764349215026, -35.75048010860329839, 2.597518595105000383 ) ) ;
#5779=CARTESIAN_POINT ( 'NONE',  ( 1.791628076902189504, -65.99651092193212776, 1.035779542278230991 ) ) ;
#5780=CARTESIAN_POINT ( 'NONE',  ( 5.575556491096470779, -57.10417477796837460, -1.782215851858570010 ) ) ;
#5790=CARTESIAN_POINT ( 'NONE',  ( 4.514859508800350696, -57.62591736726079006, 0.04509635899271501047 ) ) ;
#5792=DIRECTION ( 'NONE',  ( -0.5224671166576538850, 0.8526594349512809368, 0.000000000000000000 ) ) ;
#5794=ORIENTED_EDGE ( 'NONE', *, *, #5045, .T. ) ;
#5795=EDGE_CURVE ( 'NONE', #123, #3009, #2452, .T. ) ;
#5796=ORIENTED_EDGE ( 'NONE', *, *, #4767, .F. ) ;
#5799=CARTESIAN_POINT ( 'NONE',  ( -15.02360761328580097, -37.34705832593169816, 1.026284428608169819 ) ) ;
#5802=CARTESIAN_POINT ( 'NONE',  ( -3.697637789055789881, -65.78881948023087034, 1.221121406208630411 ) ) ;
#5803=CIRCLE ( 'NONE', #2535, 2.499999999999997335 ) ;
#5805=CARTESIAN_POINT ( 'NONE',  ( -1.110895189285712181, -65.77251424999820983, -2.870029284013874360 ) ) ;
#5806=ADVANCED_FACE ( 'NONE', ( #4188 ), #6197, .T. ) ;
#5808=SURFACE_STYLE_USAGE ( .BOTH. , #4032 ) ;
#5817=CARTESIAN_POINT ( 'NONE',  ( -2.864422359069719981, -64.63427441546140528, 2.032225693688770374 ) ) ;
#5818=AXIS2_PLACEMENT_3D ( 'NONE', #3422, #4064, #4601 ) ;
#5822=DIRECTION ( 'NONE',  ( 0.2223157560262039867, -0.6712493609847990372, 0.7071067811865450192 ) ) ;
#5823=CARTESIAN_POINT ( 'NONE',  ( 5.766865232587130130, -57.44905037028758699, 0.3380538640060152256 ) ) ;
#5824=CYLINDRICAL_SURFACE ( 'NONE', #4259, 1.000000000000000888 ) ;
#5827=VERTEX_POINT ( 'NONE', #5771 ) ;
#5828=CARTESIAN_POINT ( 'NONE',  ( -5.219056089447164481, -62.17188307074363962, 3.392373891847805467 ) ) ;
#5832=DIRECTION ( 'NONE',  ( 0.000000000000000000, 0.000000000000000000, 1.000000000000000000 ) ) ;
#5834=CARTESIAN_POINT ( 'NONE',  ( -4.908132910216119527, -63.74296424117085991, -0.6604057789239049514 ) ) ;
#5837=CARTESIAN_POINT ( 'NONE',  ( 6.187144687173720570, -58.64655194120005177, 0.3691021985165400809 ) ) ;
#5842=VERTEX_POINT ( 'NONE', #3950 ) ;
#5848=CARTESIAN_POINT ( 'NONE',  ( -3.648210298237669846, -66.52323838441711246, -0.5446899798612400145 ) ) ;
#5849=CYLINDRICAL_SURFACE ( 'NONE', #2063, 0.9999999999999984457 ) ;
#5855=CARTESIAN_POINT ( 'NONE',  ( 6.588013489872674988, -62.64654932776589646, -2.867023156876145507 ) ) ;
#5856=CARTESIAN_POINT ( 'NONE',  ( -5.524241737545620090, -57.12730840725460979, 1.694319224817255165 ) ) ;
#5857=CARTESIAN_POINT ( 'NONE',  ( 4.469984187763964556, -63.33186444122004843, 2.519959534738519746 ) ) ;
#5859=CYLINDRICAL_SURFACE ( 'NONE', #4807, 0.9999999999999991118 ) ;
#5860=CARTESIAN_POINT ( 'NONE',  ( -0.9067045181355430916, -66.16172987439199460, 1.193114471962507972 ) ) ;
#5865=PRODUCT_DEFINITION_CONTEXT ( 'detailed design', #2933, 'design' ) ;
#5866=CARTESIAN_POINT ( 'NONE',  ( -5.710866809226770258, -58.90547762198222870, 1.725351541085619500 ) ) ;
#5867=CARTESIAN_POINT ( 'NONE',  ( 6.265638173095489982, -61.94185186372677521, 0.5461908750427398873 ) ) ;
#5868=DIRECTION ( 'NONE',  ( 2.857391495672265093E-16, 4.793132013414519254E-17, 1.000000000000000000 ) ) ;
#5875=CARTESIAN_POINT ( 'NONE',  ( -3.079777581550224852, -54.72070545288789134, -0.1918259013367045740 ) ) ;
#5877=EDGE_LOOP ( 'NONE', ( #5902, #5903, #701, #5406, #4325, #3101 ) ) ;
#5884=CARTESIAN_POINT ( 'NONE',  ( 2.986904076224405014, -66.15109244657664078, 2.931604786918900363 ) ) ;
#5885=CARTESIAN_POINT ( 'NONE',  ( 4.371277347803607327, -55.97928041872565785, 2.299471528649866148 ) ) ;
#5887=CARTESIAN_POINT ( 'NONE',  ( -4.716938577623720263, -57.97996379370297149, -0.6608593144672147979 ) ) ;
#5889=CARTESIAN_POINT ( 'NONE',  ( 4.748085323256989732, -62.01668842780453872, -2.502390571778199568 ) ) ;
#5890=CARTESIAN_POINT ( 'NONE',  ( -4.425770051009331851, -64.17614344307862950, -0.6687802702403959909 ) ) ;
#5892=VERTEX_POINT ( 'NONE', #2256 ) ;
#5897=CARTESIAN_POINT ( 'NONE',  ( -5.211262431554310126, -59.36811747016641050, -0.7503612693867500738 ) ) ;
#5899=CARTESIAN_POINT ( 'NONE',  ( 6.162074140922939591, -62.32076522084695114, 2.666565443060120444 ) ) ;
#5902=ORIENTED_EDGE ( 'NONE', *, *, #2873, .F. ) ;
#5903=ORIENTED_EDGE ( 'NONE', *, *, #7382, .T. ) ;
#5905=FACE_OUTER_BOUND ( 'NONE', #4779, .T. ) ;
#5907=CARTESIAN_POINT ( 'NONE',  ( -5.727966693761760375, -63.15494832584334262, 1.398024598501910187 ) ) ;
#5922=CARTESIAN_POINT ( 'NONE',  ( -5.135436550704829628, -59.04801135763068487, 1.370314102932454814 ) ) ;
#5927=CARTESIAN_POINT ( 'NONE',  ( -5.562592810569134905, -62.20808427580125510, -0.5376115902277359693 ) ) ;
#5928=CARTESIAN_POINT ( 'NONE',  ( -1.409024882572649906, -54.10038288851608712, -0.1041033434293599513 ) ) ;
#5930=AXIS2_PLACEMENT_3D ( 'NONE', #1658, #4609, #6739 ) ;
#5933=AXIS2_PLACEMENT_3D ( 'NONE', #1422, #6701, #4901 ) ;
#5936=CARTESIAN_POINT ( 'NONE',  ( 5.465222000274489567, -57.03231251543625291, 0.2812537129946697800 ) ) ;
#5938=CARTESIAN_POINT ( 'NONE',  ( -5.207248779674009675, -62.02473276930714263, -2.515586951106906444 ) ) ;
#5942=( GEOMETRIC_REPRESENTATION_CONTEXT ( 3 ) GLOBAL_UNCERTAINTY_ASSIGNED_CONTEXT ( ( #3582 ) ) GLOBAL_UNIT_ASSIGNED_CONTEXT ( ( #2815, #2771, #78 ) ) REPRESENTATION_CONTEXT ( 'NONE', 'WORKASPACE' ) );
#5952=CARTESIAN_POINT ( 'NONE',  ( -5.253023064401910247, -61.29850624113154822, 1.730934016304810363 ) ) ;
#5954=ORIENTED_EDGE ( 'NONE', *, *, #7247, .F. ) ;
#5958=AXIS2_PLACEMENT_3D ( 'NONE', #180, #6048, #6630 ) ;
#5959=CARTESIAN_POINT ( 'NONE',  ( 0.000000000000000000, 0.000000000000000000, 0.000000000000000000 ) ) ;
#5960=DIRECTION ( 'NONE',  ( 0.3144066910790611624, 0.9492883822130744331, 6.800116025829053242E-16 ) ) ;
#5965=ORIENTED_EDGE ( 'NONE', *, *, #2721, .T. ) ;
#5968=CARTESIAN_POINT ( 'NONE',  ( 1.218291106157554093, -66.23251464141941369, 3.139314518440670110 ) ) ;
#5971=CARTESIAN_POINT ( 'NONE',  ( -0.9457358914118852988, -66.20977737079573444, -0.9048510307158501575 ) ) ;
#5975=ADVANCED_FACE ( 'NONE', ( #6931 ), #539, .T. ) ;
#5976=CARTESIAN_POINT ( 'NONE',  ( 9.311407240687648468, -51.41373841511902043, -1.002481404894999928 ) ) ;
#5984=ADVANCED_FACE ( 'NONE', ( #3036 ), #4144, .T. ) ;
#5987=CARTESIAN_POINT ( 'NONE',  ( -5.207248779674009675, -62.02473276930714263, -2.515586951106906444 ) ) ;
#5988=VERTEX_POINT ( 'NONE', #1249 ) ;
#5989=ORIENTED_EDGE ( 'NONE', *, *, #3425, .T. ) ;
#5994=CARTESIAN_POINT ( 'NONE',  ( 4.908910890503494606, -62.05094255708826978, -1.931865236676712838 ) ) ;
#5995=CARTESIAN_POINT ( 'NONE',  ( -6.093803043304910183, -63.45548452497258296, 3.342215352752540447 ) ) ;
#5996=EDGE_LOOP ( 'NONE', ( #2883, #4293, #3243, #67, #3454, #2727 ) ) ;
#5999=CARTESIAN_POINT ( 'NONE',  ( 5.463696144088109996, -62.30361170774578028, -3.475027489484119769 ) ) ;
#6000=CARTESIAN_POINT ( 'NONE',  ( -1.315849457849963988, -65.60036621133420454, 0.8401019477754300135 ) ) ;
#6001=LINE ( 'NONE', #4376, #1907 ) ;
#6002=CARTESIAN_POINT ( 'NONE',  ( 0.4753047092618455927, -54.67404102287693490, 0.1178634422923512670 ) ) ;
#6009=CARTESIAN_POINT ( 'NONE',  ( 3.403992074353090036, -54.97443010399496899, 2.224669212202579960 ) ) ;
#6010=CARTESIAN_POINT ( 'NONE',  ( -6.752862897928530117, -62.17267392066884213, 1.309913053057485177 ) ) ;
#6012=DIRECTION ( 'NONE',  ( 1.000000000000000000, 0.000000000000000000, 0.000000000000000000 ) ) ;
#6018=AXIS2_PLACEMENT_3D ( 'NONE', #683, #3001, #1848 ) ;
#6020=CARTESIAN_POINT ( 'NONE',  ( 4.520351875826989385, -63.47384446676466752, 0.9302720625520102260 ) ) ;
#6021=CARTESIAN_POINT ( 'NONE',  ( -2.400689227110559987, -66.32592643012861799, 1.119566937203962276 ) ) ;
#6025=VERTEX_POINT ( 'NONE', #80 ) ;
#6026=AXIS2_PLACEMENT_3D ( 'NONE', #4500, #2743, #6819 ) ;
#6033=CARTESIAN_POINT ( 'NONE',  ( 6.131131505788760094, -57.13037711201883440, 2.282642250695309905 ) ) ;
#6038=CARTESIAN_POINT ( 'NONE',  ( -1.747150726250749964, -54.79256248330700174, -0.04158717877314997702 ) ) ;
#6039=DIRECTION ( 'NONE',  ( -0.4328040977884316520, 0.5819352847797604200, 0.6884997728872834788 ) ) ;
#6041=CARTESIAN_POINT ( 'NONE',  ( -5.772955398150772410, -60.86632288506189070, -0.4588952161651880246 ) ) ;
#6047=CARTESIAN_POINT ( 'NONE',  ( -14.63712380658832046, -35.33334692323139592, -3.626931576674818025 ) ) ;
#6048=DIRECTION ( 'NONE',  ( 0.3144066910790611624, 0.9492883822130744331, 6.800116025829053242E-16 ) ) ;
#6049=CARTESIAN_POINT ( 'NONE',  ( 1.414957918137925930, -67.26958221326191278, 2.900267041832249593 ) ) ;
#6051=CIRCLE ( 'NONE', #6998, 1.000000000000001110 ) ;
#6052=CIRCLE ( 'NONE', #2303, 0.4999999999999991118 ) ;
#6055=ORIENTED_EDGE ( 'NONE', *, *, #669, .F. ) ;
#6060=CARTESIAN_POINT ( 'NONE',  ( -4.816289696271150333, -61.50450503696147564, 2.285640538916479780 ) ) ;
#6063=CARTESIAN_POINT ( 'NONE',  ( -2.881623215960232631, -54.84435829741126867, -0.2178263081526286560 ) ) ;
#6076=CARTESIAN_POINT ( 'NONE',  ( 3.059030343303239974, -54.77303090793805040, 0.1039292770420399137 ) ) ;
#6077=VERTEX_POINT ( 'NONE', #4676 ) ;
#6080=DIRECTION ( 'NONE',  ( 0.3128416502900970286, -0.9445788350777319931, 0.09950339776592319330 ) ) ;
#6082=CARTESIAN_POINT ( 'NONE',  ( 5.216904734083789741, -62.90507476914316953, -1.366939949738901872 ) ) ;
#6089=DIRECTION ( 'NONE',  ( 0.9492899500389727629, 0.3144019573014849023, 0.000000000000000000 ) ) ;
#6093=CARTESIAN_POINT ( 'NONE',  ( 6.775879105374429834, -62.07729961717699041, 0.4273099905340951299 ) ) ;
#6094=CARTESIAN_POINT ( 'NONE',  ( 4.748085323256989732, -62.01668842780453872, -2.502390571778199568 ) ) ;
#6100=CARTESIAN_POINT ( 'NONE',  ( 2.734303695691099989, -65.14978033110251943, -1.014598242344157963 ) ) ;
#6102=CARTESIAN_POINT ( 'NONE',  ( 0.07924247749816264175, -66.69181187827942381, 3.086254127763143895 ) ) ;
#6103=CARTESIAN_POINT ( 'NONE',  ( -5.466570931786790766, -63.95713299600960511, -2.842748680216657942 ) ) ;
#6104=ORIENTED_EDGE ( 'NONE', *, *, #2956, .T. ) ;
#6112=CARTESIAN_POINT ( 'NONE',  ( 5.465222000274489567, -57.03231251543625291, 0.2812537129946697800 ) ) ;
#6117=CARTESIAN_POINT ( 'NONE',  ( 5.267626090836840191, -63.86700364562991439, -1.442031773567929775 ) ) ;
#6118=PLANE ( 'NONE',  #2396 ) ;
#6120=EDGE_CURVE ( 'NONE', #354, #6909, #2932, .T. ) ;
#6121=ORIENTED_EDGE ( 'NONE', *, *, #738, .F. ) ;
#6126=CARTESIAN_POINT ( 'NONE',  ( 2.082020516433249924, -53.40759131075155608, 1.446381639928540297 ) ) ;
#6128=ORIENTED_EDGE ( 'NONE', *, *, #4253, .T. ) ;
#6132=CARTESIAN_POINT ( 'NONE',  ( 2.466033592522905327, -56.00841680802438560, -1.148886392136307943 ) ) ;
#6134=CARTESIAN_POINT ( 'NONE',  ( -2.343653935680388933, -66.35127301696434188, 3.217364074058102652 ) ) ;
#6143=CARTESIAN_POINT ( 'NONE',  ( 3.318166867071405068, -54.31318850506334428, -0.01554017946999016950 ) ) ;
#6147=CARTESIAN_POINT ( 'NONE',  ( 9.358334193258830425, -51.27205182843857045, -2.495037190209989930 ) ) ;
#6149=CARTESIAN_POINT ( 'NONE',  ( 4.841738599488129680, -63.57854475872899513, -1.322671891113719855 ) ) ;
#6158=FACE_OUTER_BOUND ( 'NONE', #3901, .T. ) ;
#6159=CARTESIAN_POINT ( 'NONE',  ( -5.640317424943829927, -64.23513207997909547, 3.298613272382739936 ) ) ;
#6167=CARTESIAN_POINT ( 'NONE',  ( -4.954937549494499827, -61.85628170826059602, 3.287035460711430268 ) ) ;
#6171=CARTESIAN_POINT ( 'NONE',  ( 5.248671903609490208, -63.99330799355751509, -3.505550301244489741 ) ) ;
#6179=CARTESIAN_POINT ( 'NONE',  ( 6.251545776960879763, -56.60079747432034480, -0.4089935619396500299 ) ) ;
#6185=CARTESIAN_POINT ( 'NONE',  ( 5.676184037656430093, -63.13711808556965366, -1.485967351095627720 ) ) ;
#6197=TOROIDAL_SURFACE ( 'NONE', #1263, 1.500000000000000000, 1.000000000000000000 ) ;
#6198=CARTESIAN_POINT ( 'NONE',  ( -6.487383171013251015, -57.01613561570176358, -1.117195879216653864 ) ) ;
#6204=CARTESIAN_POINT ( 'NONE',  ( -1.607783425601855054, -65.25734987882880489, 1.942476202525789342 ) ) ;
#6207=CARTESIAN_POINT ( 'NONE',  ( 4.447965418036755381, -62.61493371638615457, -2.739923498411994451 ) ) ;
#6211=EDGE_CURVE ( 'NONE', #1508, #4174, #1856, .T. ) ;
#6219=CARTESIAN_POINT ( 'NONE',  ( 3.357456528971034970, -66.96770758659590683, 2.241359037429140333 ) ) ;
#6223=CARTESIAN_POINT ( 'NONE',  ( -6.129265975028279634, -62.42766041111902098, -0.6909925287373350766 ) ) ;
#6229=CARTESIAN_POINT ( 'NONE',  ( -5.480856739662490540, -62.25220485324549458, 1.560007870815685260 ) ) ;
#6230=EDGE_CURVE ( 'NONE', #2342, #6356, #2817, .T. ) ;
#6232=CARTESIAN_POINT ( 'NONE',  ( -7.175161506198990402, -58.91160695923000645, -1.204451995733903935 ) ) ;
#6236=CARTESIAN_POINT ( 'NONE',  ( 1.460134286533229853, -55.58368472982129305, 0.8822880931559249351 ) ) ;
#6237=DIRECTION ( 'NONE',  ( 0.1860016876085203441, -0.1636620475539279917, 0.9688230521603200529 ) ) ;
#6242=CARTESIAN_POINT ( 'NONE',  ( 0.002312830554035623463, -66.69201937025515292, -1.109451928479881833 ) ) ;
#6246=ORIENTED_EDGE ( 'NONE', *, *, #2365, .F. ) ;
#6250=CYLINDRICAL_SURFACE ( 'NONE', #1843, 1.000000000000000888 ) ;
#6252=CARTESIAN_POINT ( 'NONE',  ( 7.059059989562619819, -58.43975188330606585, -0.3221438859163246460 ) ) ;
#6253=TOROIDAL_SURFACE ( 'NONE', #6018, 1.500000000000000000, 1.000000000000000000 ) ;
#6254=FACE_OUTER_BOUND ( 'NONE', #6634, .T. ) ;
#6255=DIRECTION ( 'NONE',  ( 0.2164621326156030423, -0.07169280077033016174, 0.9736551173085935540 ) ) ;
#6268=CARTESIAN_POINT ( 'NONE',  ( 1.647105754412080181, -53.29316706828264216, -0.6741030570719998005 ) ) ;
#6273=CARTESIAN_POINT ( 'NONE',  ( -5.121204309455420045, -61.36711808260334067, 3.320501707867800523 ) ) ;
#6277=CARTESIAN_POINT ( 'NONE',  ( 2.751515497641074948, -64.99867735210931130, 0.5749532485596650089 ) ) ;
#6280=AXIS2_PLACEMENT_3D ( 'NONE', #6565, #1405, #4882 ) ;
#6288=CARTESIAN_POINT ( 'NONE',  ( -6.429839020462739363, -63.58404662519255623, 2.770540757372710328 ) ) ;
#6306=AXIS2_PLACEMENT_3D ( 'NONE', #2282, #144, #1875 ) ;
#6311=CARTESIAN_POINT ( 'NONE',  ( 6.738276468386390050, -62.65933952543014129, -2.221138621355481568 ) ) ;
#6317=CARTESIAN_POINT ( 'NONE',  ( -5.163597282883630513, -63.01551968439245144, 3.580859834736030312 ) ) ;
#6321=ORIENTED_EDGE ( 'NONE', *, *, #339, .T. ) ;
#6326=CARTESIAN_POINT ( 'NONE',  ( -9.311346830843410416, -51.41373841511902043, 3.533728595105000370 ) ) ;
#6327=CARTESIAN_POINT ( 'NONE',  ( -6.026503769217380402, -56.70691413961192495, -0.01483612153302480557 ) ) ;
#6328=CARTESIAN_POINT ( 'NONE',  ( -5.788105944719140084, -64.22553544194731501, 1.709038299673605321 ) ) ;
#6337=ADVANCED_FACE ( 'NONE', ( #1614 ), #6250, .T. ) ;
#6345=CARTESIAN_POINT ( 'NONE',  ( 6.291895255447879975, -62.07086823355334104, -1.517278733858541839 ) ) ;
#6351=CARTESIAN_POINT ( 'NONE',  ( -1.095027572700850049, -66.25608112803911354, -0.9253912358714898589 ) ) ;
#6355=VERTEX_POINT ( 'NONE', #1571 ) ;
#6356=VERTEX_POINT ( 'NONE', #2808 ) ;
#6357=ORIENTED_EDGE ( 'NONE', *, *, #2035, .F. ) ;
#6358=CARTESIAN_POINT ( 'NONE',  ( -15.02360761328580097, -37.34705832593169816, 1.026284428608169819 ) ) ;
#6360=CARTESIAN_POINT ( 'NONE',  ( 6.364381519408680354, -59.13673167413750775, 0.4262454961123699482 ) ) ;
#6362=CARTESIAN_POINT ( 'NONE',  ( -2.818432829560444830, -65.09919931551695527, -0.6601304211325950133 ) ) ;
#6369=CARTESIAN_POINT ( 'NONE',  ( 5.661113010068490325, -57.37064013373739613, 2.401523511004880262 ) ) ;
#6372=DIRECTION ( 'NONE',  ( 2.290931512739800066E-16, 1.403768413105889815E-16, 1.000000000000000000 ) ) ;
#6374=CARTESIAN_POINT ( 'NONE',  ( 4.121185724914560033, -64.58760431682401304, 0.8784256758975720336 ) ) ;
#6379=EDGE_CURVE ( 'NONE', #1750, #2698, #6535, .T. ) ;
#6384=CARTESIAN_POINT ( 'NONE',  ( 5.677676720488819662, -58.78440004686129328, 0.4885712913175552785 ) ) ;
#6385=CARTESIAN_POINT ( 'NONE',  ( -3.498019654714389581, -55.03494779767484602, -0.2490962732230048438 ) ) ;
#6396=CARTESIAN_POINT ( 'NONE',  ( -6.338727533122220592, -59.01378846946391832, -2.577673957235475211 ) ) ;
#6401=DIRECTION ( 'NONE',  ( -0.9492899500389727629, -0.3144019573014849023, 0.000000000000000000 ) ) ;
#6405=CARTESIAN_POINT ( 'NONE',  ( -1.592557218785495055, -66.68601476236933934, 1.076257986235874764 ) ) ;
#6409=CARTESIAN_POINT ( 'NONE',  ( -2.954381708604445045, -64.87272166844897470, 3.050067095118260241 ) ) ;
#6412=STYLED_ITEM ( 'NONE', ( #6847 ), #7333 ) ;
#6415=CARTESIAN_POINT ( 'NONE',  ( 6.364381519408680354, -59.13673167413750775, 0.4262454961123699482 ) ) ;
#6417=DIRECTION ( 'NONE',  ( 0.2223157560262043198, -0.6712493609847984821, 0.7071067811865453523 ) ) ;
#6423=CARTESIAN_POINT ( 'NONE',  ( 1.218291106157554093, -66.23251464141941369, 3.139314518440670110 ) ) ;
#6425=CARTESIAN_POINT ( 'NONE',  ( 1.402950248545461909, -54.15620739517822813, 0.01614447287717020105 ) ) ;
#6428=EDGE_CURVE ( 'NONE', #7272, #1033, #408, .T. ) ;
#6434=CARTESIAN_POINT ( 'NONE',  ( -6.176129832103540274, -61.75772637036916279, 1.476179264717100370 ) ) ;
#6444=CARTESIAN_POINT ( 'NONE',  ( 1.990789772983897477, -66.41826147249288681, 0.8834450765732816402 ) ) ;
#6445=CARTESIAN_POINT ( 'NONE',  ( 5.257784700090706309, -62.23303559029498899, -3.424757160461740835 ) ) ;
#6447=CARTESIAN_POINT ( 'NONE',  ( -1.721951098409294945, -66.71030961465282871, -0.9872116442447198548 ) ) ;
#6449=DIRECTION ( 'NONE',  ( 0.3128463504745285229, 0.9445772445362839997, 0.09950371902099811039 ) ) ;
#6451=DIRECTION ( 'NONE',  ( 0.2164621326156030423, -0.07169280077033016174, 0.9736551173085935540 ) ) ;
#6453=CARTESIAN_POINT ( 'NONE',  ( -1.397697773942189858, -54.69607029038206747, 2.078897745975250455 ) ) ;
#6454=CARTESIAN_POINT ( 'NONE',  ( 5.676184037656430093, -63.13711808556965366, -1.485967351095627720 ) ) ;
#6462=CARTESIAN_POINT ( 'NONE',  ( 14.97072768011073940, -34.32654753528365177, 2.597518595105000383 ) ) ;
#6463=CARTESIAN_POINT ( 'NONE',  ( -1.721951098409294945, -66.71030961465282871, -0.9872116442447198548 ) ) ;
#6464=CARTESIAN_POINT ( 'NONE',  ( 6.643375263299909683, -62.64442119333418901, -2.502572238011808281 ) ) ;
#6467=DIRECTION ( 'NONE',  ( 1.000000000000000000, 0.000000000000000000, 0.000000000000000000 ) ) ;
#6468=EDGE_CURVE ( 'NONE', #1675, #7067, #571, .T. ) ;
#6474=CARTESIAN_POINT ( 'NONE',  ( 2.533447467746755333, -55.76293992159236979, -0.1309777151760100067 ) ) ;
#6476=CARTESIAN_POINT ( 'NONE',  ( -0.8826897099904034150, -54.72534079625300052, 0.03922796265859054832 ) ) ;
#6477=CARTESIAN_POINT ( 'NONE',  ( 6.493768279116130415, -62.63809584774485018, -3.239169643854469705 ) ) ;
#6479=DIRECTION ( 'NONE',  ( -0.2467992669038191755, 0.02032136184815236737, 0.9688535307818070264 ) ) ;
#6483=CARTESIAN_POINT ( 'NONE',  ( 1.785462125252589960, -54.25404267560509908, 2.136629312307830375 ) ) ;
#6484=CARTESIAN_POINT ( 'NONE',  ( -4.614416121558960526, -57.55752852796073427, -0.1302737383155048445 ) ) ;
#6487=CARTESIAN_POINT ( 'NONE',  ( 15.08188723176695056, -33.99092340910145538, 5.072392329257909616 ) ) ;
#6488=ORIENTED_EDGE ( 'NONE', *, *, #1862, .T. ) ;
#6489=PRODUCT_DEFINITION ( 'UNKNOWN', '', #159, #5865 ) ;
#6490=VERTEX_POINT ( 'NONE', #2370 ) ;
#6494=CARTESIAN_POINT ( 'NONE',  ( -1.435618805647706164, -65.69410370267330279, -0.7494494782121799981 ) ) ;
#6495=CARTESIAN_POINT ( 'NONE',  ( 6.133675886466185112, -62.42807403084368900, -1.580205649328261241 ) ) ;
#6496=CIRCLE ( 'NONE', #3973, 1.000000000000001110 ) ;
#6500=EDGE_LOOP ( 'NONE', ( #1301, #4370, #5297, #7126, #2925, #3282 ) ) ;
#6504=CARTESIAN_POINT ( 'NONE',  ( -5.628700163094269016, -63.23550210468251009, 3.461537593744290042 ) ) ;
#6510=CARTESIAN_POINT ( 'NONE',  ( -4.773669824303439668, -63.68048849998092464, 3.536592896228280214 ) ) ;
#6514=CARTESIAN_POINT ( 'NONE',  ( -1.329205950148755644, -54.81433347601338113, 0.01301773866004049540 ) ) ;
#6519=TOROIDAL_SURFACE ( 'NONE', #5818, 1.500000000000000000, 1.000000000000000000 ) ;
#6526=CARTESIAN_POINT ( 'NONE',  ( -3.235261603508409856, -66.01500717273368934, 1.164464255201294929 ) ) ;
#6527=DIRECTION ( 'NONE',  ( 0.2223191033124283789, 0.6712482523644727195, 0.7071067811865466846 ) ) ;
#6528=ORIENTED_EDGE ( 'NONE', *, *, #6379, .T. ) ;
#6533=VECTOR ( 'NONE', #3173, 1000.000000000000000 ) ;
#6534=CYLINDRICAL_SURFACE ( 'NONE', #4623, 0.9999999999999980016 ) ;
#6535=CIRCLE ( 'NONE', #5228, 1.000000000000001776 ) ;
#6537=CARTESIAN_POINT ( 'NONE',  ( 3.594547628745600409, -65.86039197651267330, -3.372550074330296965 ) ) ;
#6548=CARTESIAN_POINT ( 'NONE',  ( -6.026198395890769888, -63.94474587426248036, 1.222360836057740041 ) ) ;
#6549=ORIENTED_EDGE ( 'NONE', *, *, #38, .T. ) ;
#6552=CARTESIAN_POINT ( 'NONE',  ( 2.799893819535080208, -55.23287331081275653, 0.2233987335540700003 ) ) ;
#6553=ADVANCED_FACE ( 'NONE', ( #6961 ), #1956, .T. ) ;
#6556=CARTESIAN_POINT ( 'NONE',  ( -6.629462435860018488, -62.64420580508557634, 2.974566524362353803 ) ) ;
#6557=CARTESIAN_POINT ( 'NONE',  ( 5.463696144088109996, -62.30361170774578028, -3.475027489484119769 ) ) ;
#6559=CARTESIAN_POINT ( 'NONE',  ( -13.49899450467539985, -35.75040780681265318, -2.566271404894997499 ) ) ;
#6563=CARTESIAN_POINT ( 'NONE',  ( -5.714251477591489881, -57.46902543231049521, -0.4259505751857597389 ) ) ;
#6564=CARTESIAN_POINT ( 'NONE',  ( -2.148471732745839802, -67.07461398899560834, 3.078016402823839925 ) ) ;
#6565=CARTESIAN_POINT ( 'NONE',  ( -14.02739156872318027, -37.17434273187110705, -0.4662714048949997969 ) ) ;
#6568=PRODUCT_DEFINITION_SHAPE ( 'NONE', 'NONE',  #6489 ) ;
#6572=CARTESIAN_POINT ( 'NONE',  ( -4.461725341067024786, -62.58642870417541104, 2.208339520507450082 ) ) ;
#6573=CARTESIAN_POINT ( 'NONE',  ( -0.01776538050268356914, -54.19622611322429862, -0.06040963844522982684 ) ) ;
#6574=ORIENTED_EDGE ( 'NONE', *, *, #5421, .T. ) ;
#6579=DIRECTION ( 'NONE',  ( -0.2467992669038191478, 0.02032136184815930280, 0.9688535307818069153 ) ) ;
#6580=CARTESIAN_POINT ( 'NONE',  ( -3.403807323753265113, -54.36107883567960641, 1.752763223655470437 ) ) ;
#6584=CARTESIAN_POINT ( 'NONE',  ( 5.010558598472139913, -57.30068827582834956, 0.4001341763009204078 ) ) ;
#6586=CARTESIAN_POINT ( 'NONE',  ( -5.904042796847299712, -62.42803713013675093, 3.506543003539000392 ) ) ;
#6587=CARTESIAN_POINT ( 'NONE',  ( 5.724602046902682595, -59.58971228651716245, -1.534163154136720442 ) ) ;
#6590=DIRECTION ( 'NONE',  ( -0.9492899500389725409, -0.3144019573014856794, 0.000000000000000000 ) ) ;
#6591=DIRECTION ( 'NONE',  ( 0.9492883822130744331, -0.3144066910790611624, 0.000000000000000000 ) ) ;
#6594=CARTESIAN_POINT ( 'NONE',  ( -1.206827191127304078, -66.77204028133226643, -1.044217440639481742 ) ) ;
#6595=CARTESIAN_POINT ( 'NONE',  ( 1.944327905822930136, -53.75057748617523856, 2.017748614706070143 ) ) ;
#6598=EDGE_CURVE ( 'NONE', #4300, #3483, #3758, .T. ) ;
#6600=ORIENTED_EDGE ( 'NONE', *, *, #2322, .F. ) ;
#6604=CARTESIAN_POINT ( 'NONE',  ( -5.227302941343250353, -58.92678856866081105, -0.2192372590660296439 ) ) ;
#6605=DIRECTION ( 'NONE',  ( -0.2467992669038191478, 0.02032136184815930280, 0.9688535307818069153 ) ) ;
#6606=CARTESIAN_POINT ( 'NONE',  ( -0.8961004093985418528, -66.62686089995901284, 3.138778905044528500 ) ) ;
#6607=EDGE_LOOP ( 'NONE', ( #508, #5415, #6973, #3319, #3943, #6600 ) ) ;
#6608=ORIENTED_EDGE ( 'NONE', *, *, #4679, .F. ) ;
#6610=CIRCLE ( 'NONE', #1909, 1.000000000000000888 ) ;
#6615=CARTESIAN_POINT ( 'NONE',  ( -6.822623972396280934, -59.02239909983155286, -0.6330850349556997880 ) ) ;
#6618=CIRCLE ( 'NONE', #5551, 1.000000000000001776 ) ;
#6620=CARTESIAN_POINT ( 'NONE',  ( -5.595710845088040841, -61.75488600311453524, 3.658668618637090031 ) ) ;
#6621=ORIENTED_EDGE ( 'NONE', *, *, #2475, .F. ) ;
#6625=FACE_OUTER_BOUND ( 'NONE', #785, .T. ) ;
#6629=CARTESIAN_POINT ( 'NONE',  ( 6.645018675491529692, -62.64496150164843158, -2.502481404895003259 ) ) ;
#6630=DIRECTION ( 'NONE',  ( 0.2164621326156030423, -0.07169280077033016174, 0.9736551173085935540 ) ) ;
#6631=CARTESIAN_POINT ( 'NONE',  ( -3.773574383489684880, -54.58470482469731877, -0.3679774332281250393 ) ) ;
#6634=EDGE_LOOP ( 'NONE', ( #292, #1496, #2586, #2121, #6982, #2759 ) ) ;
#6640=DIRECTION ( 'NONE',  ( 0.2223157560262039867, -0.6712493609847990372, 0.7071067811865450192 ) ) ;
#6643=CARTESIAN_POINT ( 'NONE',  ( -6.217266535765080704, -62.33106447713396392, -2.754524245347104383 ) ) ;
#6645=CARTESIAN_POINT ( 'NONE',  ( 2.014066015375293617, -66.41055546370263585, 2.981310916594474225 ) ) ;
#6652=SHAPE_REPRESENTATION_RELATIONSHIP ( 'NONE' , 'NONE' ,  #7047, #5592 ) ;
#6654=TOROIDAL_SURFACE ( 'NONE', #5100, 1.500000000000000000, 1.000000000000000000 ) ;
#6658=CARTESIAN_POINT ( 'NONE',  ( -5.714251477591489881, -57.46902543231049521, -0.4259505751857597389 ) ) ;
#6664=CARTESIAN_POINT ( 'NONE',  ( -1.206827191127304078, -66.77204028133226643, -1.044217440639481742 ) ) ;
#6671=CARTESIAN_POINT ( 'NONE',  ( -9.358272925367041140, -51.27205205187813419, 2.526284428608170263 ) ) ;
#6674=CARTESIAN_POINT ( 'NONE',  ( 9.389618828306289799, -51.17759410398493714, -3.490074380419979860 ) ) ;
#6676=CARTESIAN_POINT ( 'NONE',  ( -6.093803043304910183, -63.45548452497258296, 3.342215352752540447 ) ) ;
#6683=CARTESIAN_POINT ( 'NONE',  ( 1.080279179814437773, -65.65553934942860792, 2.784998920779040432 ) ) ;
#6685=CARTESIAN_POINT ( 'NONE',  ( 6.248302252609925667, -60.41094430931507020, 0.4638711834344099727 ) ) ;
#6687=CARTESIAN_POINT ( 'NONE',  ( -5.172139827190740391, -61.55016382346040871, 1.714186298074440007 ) ) ;
#6695=CARTESIAN_POINT ( 'NONE',  ( -1.626396133375414887, -53.66552156771879112, 1.839959185157149957 ) ) ;
#6701=DIRECTION ( 'NONE',  ( -0.9492883822130744331, 0.3144066910790611624, 0.000000000000000000 ) ) ;
#6702=CARTESIAN_POINT ( 'NONE',  ( 2.080482015124565098, -66.54183146390657555, -1.221303033644861813 ) ) ;
#6707=CARTESIAN_POINT ( 'NONE',  ( 14.49911764349215915, -35.75048010860329839, 0.4975185951050001831 ) ) ;
#6709=CARTESIAN_POINT ( 'NONE',  ( 6.696612653858620590, -58.50870383553881737, 0.2496331057155200817 ) ) ;
#6715=CARTESIAN_POINT ( 'NONE',  ( 2.467202665543605011, -65.15865635802147438, 2.695445654378740397 ) ) ;
#6717=CARTESIAN_POINT ( 'NONE',  ( 0.9768556859363289879, -66.61496767163153265, -1.161982190194281062 ) ) ;
#6719=ORIENTED_EDGE ( 'NONE', *, *, #4473, .T. ) ;
#6722=DIRECTION ( 'NONE',  ( 0.9492883822130744331, -0.3144066910790611624, 0.000000000000000000 ) ) ;
#6726=EDGE_CURVE ( 'NONE', #5349, #2665, #1205, .T. ) ;
#6728=CYLINDRICAL_SURFACE ( 'NONE', #4839, 1.000000000000001332 ) ;
#6730=CARTESIAN_POINT ( 'NONE',  ( 5.465222000274489567, -57.03231251543625291, 0.2812537129946697800 ) ) ;
#6739=DIRECTION ( 'NONE',  ( -0.9492883822130750993, 0.3144066910790586089, 0.000000000000000000 ) ) ;
#6740=DIRECTION ( 'NONE',  ( 0.000000000000000000, 0.000000000000000000, 1.000000000000000000 ) ) ;
#6743=CARTESIAN_POINT ( 'NONE',  ( -2.113079283527464991, -53.41662231759018198, -0.8523026345115048974 ) ) ;
#6747=CARTESIAN_POINT ( 'NONE',  ( 4.485945982887084682, -58.07227379738043993, 1.147183751133595386 ) ) ;
#6751=CARTESIAN_POINT ( 'NONE',  ( 1.460134286533229853, -55.58368472982129305, 0.8822880931559249351 ) ) ;
#6752=AXIS2_PLACEMENT_3D ( 'NONE', #3378, #5130, #7409 ) ;
#6757=VERTEX_POINT ( 'NONE', #6805 ) ;
#6763=CARTESIAN_POINT ( 'NONE',  ( 7.124841322228030904, -62.19900605811294980, -0.1440571144897197509 ) ) ;
#6764=ORIENTED_EDGE ( 'NONE', *, *, #5045, .F. ) ;
#6765=AXIS2_PLACEMENT_3D ( 'NONE', #6462, #2987, #806 ) ;
#6770=VECTOR ( 'NONE', #5832, 1000.000000000000000 ) ;
#6771=CARTESIAN_POINT ( 'NONE',  ( 3.371673436877395069, -65.30458424753078361, -1.190358958913985798 ) ) ;
#6772=AXIS2_PLACEMENT_3D ( 'NONE', #4921, #7167, #5529 ) ;
#6781=FACE_OUTER_BOUND ( 'NONE', #2423, .T. ) ;
#6784=CARTESIAN_POINT ( 'NONE',  ( 2.327488905229944560, -67.40324771348248589, -1.912586833593244773 ) ) ;
#6790=CARTESIAN_POINT ( 'NONE',  ( -4.653276882800380321, -62.74377975942224595, 3.226317067983300202 ) ) ;
#6793=CARTESIAN_POINT ( 'NONE',  ( -4.882243101556620779, -59.05916974321930724, 0.3521297881290503806 ) ) ;
#6797=CARTESIAN_POINT ( 'NONE',  ( -1.756031117750795234, -65.59594772693552045, 1.371125244074580030 ) ) ;
#6805=CARTESIAN_POINT ( 'NONE',  ( -8.362056880804429326, -51.09933645781752887, 2.533728595105000370 ) ) ;
#6806=CARTESIAN_POINT ( 'NONE',  ( 6.281284389406939894, -57.15453665621128465, 0.6930907858711948810 ) ) ;
#6809=CARTESIAN_POINT ( 'NONE',  ( -14.85943956261452037, -34.66209756224660055, -2.919824795488267455 ) ) ;
#6810=CARTESIAN_POINT ( 'NONE',  ( -6.199032880790720235, -61.56120177486793210, 3.556545127952429830 ) ) ;
#6819=DIRECTION ( 'NONE',  ( -0.08966155106958693943, -0.9959722919136836383, 0.000000000000000000 ) ) ;
#6820=CARTESIAN_POINT ( 'NONE',  ( -6.776085205154060986, -62.52991726716069820, -2.400146893717961749 ) ) ;
#6824=CARTESIAN_POINT ( 'NONE',  ( -4.882243101556620779, -59.05916974321930724, 0.3521297881290503806 ) ) ;
#6826=CARTESIAN_POINT ( 'NONE',  ( -14.02739156872318027, -37.17434273187110705, -0.4662714048949997969 ) ) ;
#6827=CARTESIAN_POINT ( 'NONE',  ( -1.315849457849963988, -65.60036621133420454, 0.8401019477754300135 ) ) ;
#6836=DIRECTION ( 'NONE',  ( 0.3128416502900965290, -0.9445788350777318820, 0.09950339776592408148 ) ) ;
#6839=DIRECTION ( 'NONE',  ( 1.000000000000000000, 0.000000000000000000, 0.000000000000000000 ) ) ;
#6841=CARTESIAN_POINT ( 'NONE',  ( -6.626722312431940765, -62.23055248060769884, 1.814117920127710226 ) ) ;
#6847=PRESENTATION_STYLE_ASSIGNMENT (( #5808 ) ) ;
#6859=CARTESIAN_POINT ( 'NONE',  ( 6.836834775951150078, -58.56388191083841122, -1.340052733437185895 ) ) ;
#6862=CARTESIAN_POINT ( 'NONE',  ( -4.803738746926375036, -62.03564609396137541, 2.885421999583970720 ) ) ;
#6866=CARTESIAN_POINT ( 'NONE',  ( 3.023925381325990092, -64.82443887782423531, -1.545558412227113765 ) ) ;
#6872=VERTEX_POINT ( 'NONE', #6989 ) ;
#6873=EDGE_LOOP ( 'NONE', ( #2138, #5417, #2364, #2812, #1344, #5072 ) ) ;
#6874=EDGE_CURVE ( 'NONE', #6757, #6490, #1765, .T. ) ;
#6882=CARTESIAN_POINT ( 'NONE',  ( -3.551508372363994859, -54.02225908916108210, 1.181396430060940306 ) ) ;
#6883=ORIENTED_EDGE ( 'NONE', *, *, #1043, .T. ) ;
#6887=FILL_AREA_STYLE ('',( #1172 ) ) ;
#6888=ADVANCED_FACE ( 'NONE', ( #6926 ), #5849, .T. ) ;
#6893=CARTESIAN_POINT ( 'NONE',  ( 6.419789085491157898, -62.60659963283899998, -3.157657936188097203 ) ) ;
#6896=( GEOMETRIC_REPRESENTATION_CONTEXT ( 3 ) GLOBAL_UNCERTAINTY_ASSIGNED_CONTEXT ( ( #2072 ) ) GLOBAL_UNIT_ASSIGNED_CONTEXT ( ( #5276, #367, #4362 ) ) REPRESENTATION_CONTEXT ( 'NONE', 'WORKASPACE' ) );
#6905=DIRECTION ( 'NONE',  ( 0.000000000000000000, -0.7252570966694443788, 0.6884781359858918037 ) ) ;
#6906=CARTESIAN_POINT ( 'NONE',  ( -3.648210298237669846, -66.52323838441711246, -0.5446899798612400145 ) ) ;
#6909=VERTEX_POINT ( 'NONE', #4092 ) ;
#6911=CARTESIAN_POINT ( 'NONE',  ( 14.63724902514211834, -35.33341991383040437, 3.658178766884810251 ) ) ;
#6915=CARTESIAN_POINT ( 'NONE',  ( 5.755397240816559901, -61.80640411027656000, 0.6650717595513898628 ) ) ;
#6917=DIRECTION ( 'NONE',  ( -0.9492883822130750993, 0.3144066910790588865, 0.000000000000000000 ) ) ;
#6921=VERTEX_POINT ( 'NONE', #3417 ) ;
#6924=CARTESIAN_POINT ( 'NONE',  ( 5.927764221498110331, -62.35749858221746678, -1.529935281190306862 ) ) ;
#6925=CARTESIAN_POINT ( 'NONE',  ( 5.766865232587130130, -57.44905037028758699, 0.3380538640060152256 ) ) ;
#6926=FACE_OUTER_BOUND ( 'NONE', #1644, .T. ) ;
#6927=CARTESIAN_POINT ( 'NONE',  ( 4.666229687490379696, -57.64092629874981810, -1.544454925248829991 ) ) ;
#6931=FACE_OUTER_BOUND ( 'NONE', #1793, .T. ) ;
#6937=ORIENTED_EDGE ( 'NONE', *, *, #5043, .T. ) ;
#6938=DIRECTION ( 'NONE',  ( -0.3144019573014875113, 0.9492899500389717637, 0.000000000000000000 ) ) ;
#6943=CARTESIAN_POINT ( 'NONE',  ( -5.032169712422947860, -62.11039060171678017, 3.232780297333488040 ) ) ;
#6946=CARTESIAN_POINT ( 'NONE',  ( -9.311346830843410416, -51.41373841511902043, 2.533728595105000370 ) ) ;
#6947=CARTESIAN_POINT ( 'NONE',  ( 5.113035703684060351, -58.96629286118465529, 0.1341944340671852032 ) ) ;
#6948=CARTESIAN_POINT ( 'NONE',  ( -5.563801105733269914, -63.69014839564722763, 1.341242183458755344 ) ) ;
#6953=CARTESIAN_POINT ( 'NONE',  ( -3.427937952159080037, -54.92350006295870202, -2.312565912944844371 ) ) ;
#6961=FACE_OUTER_BOUND ( 'NONE', #3181, .T. ) ;
#6962=CARTESIAN_POINT ( 'NONE',  ( 1.785462125252589960, -54.25404267560509908, 2.136629312307830375 ) ) ;
#6964=CARTESIAN_POINT ( 'NONE',  ( -4.470547512179178895, -58.04376326654274720, -1.678768375691622960 ) ) ;
#6973=ORIENTED_EDGE ( 'NONE', *, *, #3082, .T. ) ;
#6976=AXIS2_PLACEMENT_3D ( 'NONE', #2775, #3309, #378 ) ;
#6978=CARTESIAN_POINT ( 'NONE',  ( -4.716938577623720263, -57.97996379370297149, -0.6608593144672147979 ) ) ;
#6979=CARTESIAN_POINT ( 'NONE',  ( -5.628700163094269016, -63.23550210468251009, 3.461537593744290042 ) ) ;
#6982=ORIENTED_EDGE ( 'NONE', *, *, #1180, .F. ) ;
#6986=EDGE_CURVE ( 'NONE', #3009, #1758, #4983, .T. ) ;
#6988=CARTESIAN_POINT ( 'NONE',  ( 6.871427970997950219, -62.19563859352643931, -1.162241389626079702 ) ) ;
#6989=CARTESIAN_POINT ( 'NONE',  ( -14.18459254737392072, -36.69969775685165558, -2.566271404894997499 ) ) ;
#6997=CARTESIAN_POINT ( 'NONE',  ( 2.808545138791364693, -54.80713269388122200, 2.194622045337712102 ) ) ;
#6998=AXIS2_PLACEMENT_3D ( 'NONE', #866, #7156, #1995 ) ;
#6999=CARTESIAN_POINT ( 'NONE',  ( 5.178445921634760474, -62.11857673748845343, 0.8408583081513953950 ) ) ;
#7002=CARTESIAN_POINT ( 'NONE',  ( -4.663084970140659813, -61.97199652813008441, 2.252239320826900482 ) ) ;
#7005=CARTESIAN_POINT ( 'NONE',  ( 2.672475618906553940, -55.25697960364365713, 0.2490731612973094422 ) ) ;
#7006=CARTESIAN_POINT ( 'NONE',  ( -5.509265921604280081, -56.99747518668161206, -0.3692125993829896702 ) ) ;
#7009=ORIENTED_EDGE ( 'NONE', *, *, #5043, .F. ) ;
#7017=CARTESIAN_POINT ( 'NONE',  ( 5.447354608442940282, -62.18425133612383604, -1.411124226719259855 ) ) ;
#7023=EDGE_CURVE ( 'NONE', #2665, #1675, #5052, .T. ) ;
#7030=CARTESIAN_POINT ( 'NONE',  ( 6.134453413605339911, -63.99854120705014537, -1.074823505768055742 ) ) ;
#7040=CARTESIAN_POINT ( 'NONE',  ( 3.116905194451685013, -55.41725085606579171, 2.344137946175070653 ) ) ;
#7041=DIRECTION ( 'NONE',  ( 0.9492899500389725409, 0.3144019573014856794, 0.000000000000000000 ) ) ;
#7044=DIRECTION ( 'NONE',  ( 0.1860016876085203719, -0.1636620475539280195, 0.9688230521603200529 ) ) ;
#7045=CARTESIAN_POINT ( 'NONE',  ( -6.079305786110669629, -62.05959118544440400, 1.459294228111509995 ) ) ;
#7047=SHAPE_REPRESENTATION ( 'Return Torsion Spring', ( #751 ), #6896 ) ;
#7052=CARTESIAN_POINT ( 'NONE',  ( -5.996378862946620814, -62.15612413928192836, 3.522786485084270058 ) ) ;
#7053=CARTESIAN_POINT ( 'NONE',  ( 2.671142801832544933, -55.70169962949673703, -1.720663637103989618 ) ) ;
#7055=DIRECTION ( 'NONE',  ( -0.5224671166576538850, 0.8526594349512809368, 0.000000000000000000 ) ) ;
#7064=CARTESIAN_POINT ( 'NONE',  ( 6.272193759149150338, -58.74577472516177323, -1.694429590687548837 ) ) ;
#7067=VERTEX_POINT ( 'NONE', #5999 ) ;
#7072=CARTESIAN_POINT ( 'NONE',  ( 1.159215146223531834, -55.24985087088717250, -0.2200125624336850272 ) ) ;
#7074=CARTESIAN_POINT ( 'NONE',  ( -5.480856739662490540, -62.25220485324549458, 1.560007870815685260 ) ) ;
#7075=CARTESIAN_POINT ( 'NONE',  ( 5.174390334401523184, -63.14351876211269854, -1.324289845673988442 ) ) ;
#7076=CARTESIAN_POINT ( 'NONE',  ( -5.671911954242359499, -63.61502870002530585, -0.7222274751851948116 ) ) ;
#7079=AXIS2_PLACEMENT_3D ( 'NONE', #5483, #3158, #3193 ) ;
#7084=CARTESIAN_POINT ( 'NONE',  ( -6.199032880790720235, -61.56120177486793210, 3.556545127952429830 ) ) ;
#7089=CARTESIAN_POINT ( 'NONE',  ( 10.30762257547189975, -51.58645851951763461, -2.495037190209991707 ) ) ;
#7091=CARTESIAN_POINT ( 'NONE',  ( 1.014503381694089823, -65.79094358639915185, 1.195300268011630029 ) ) ;
#7098=DIRECTION ( 'NONE',  ( 0.1860016876085203719, -0.1636620475539280195, 0.9688230521603200529 ) ) ;
#7099=CARTESIAN_POINT ( 'NONE',  ( 4.781940407807399929, -62.01839479521094489, -2.202197501157848958 ) ) ;
#7100=CARTESIAN_POINT ( 'NONE',  ( -5.354034084503060065, -64.02545556441495478, -0.7792797212839647214 ) ) ;
#7106=CARTESIAN_POINT ( 'NONE',  ( -2.909477865675369923, -55.29415281518058833, 1.990524098341705406 ) ) ;
#7111=CARTESIAN_POINT ( 'NONE',  ( 0.8643374975182065434, -66.22190918914451174, -1.009590967482013601 ) ) ;
#7112=EDGE_LOOP ( 'NONE', ( #5794, #5723 ) ) ;
#7115=AXIS2_PLACEMENT_3D ( 'NONE', #3034, #296, #5353 ) ;
#7120=VECTOR ( 'NONE', #6640, 1000.000000000000114 ) ;
#7122=CARTESIAN_POINT ( 'NONE',  ( -3.569041007005829602, -65.81017109676685095, 3.284668648760890264 ) ) ;
#7124=CARTESIAN_POINT ( 'NONE',  ( -5.957512881900739465, -64.40555820178136059, 2.727170671215090270 ) ) ;
#7126=ORIENTED_EDGE ( 'NONE', *, *, #4905, .T. ) ;
#7130=CIRCLE ( 'NONE', #24, 1.000000000000000000 ) ;
#7134=CARTESIAN_POINT ( 'NONE',  ( 4.697834216849050115, -63.19072998194386059, -1.190263883463073880 ) ) ;
#7136=CARTESIAN_POINT ( 'NONE',  ( 6.002340677743171149, -62.35123097424496308, 0.5688650469685809785 ) ) ;
#7144=CARTESIAN_POINT ( 'NONE',  ( 6.265638173095489982, -61.94185186372677521, 0.5461908750427398873 ) ) ;
#7149=CARTESIAN_POINT ( 'NONE',  ( 4.689255334142830023, -62.66924379293478609, -1.721810340931042793 ) ) ;
#7151=DIRECTION ( 'NONE',  ( 0.3144019573014849023, -0.9492899500389727629, 0.000000000000000000 ) ) ;
#7152=EDGE_CURVE ( 'NONE', #1826, #4852, #1374, .T. ) ;
#7153=CARTESIAN_POINT ( 'NONE',  ( 2.694291810223862882, -55.26708005044292094, -1.848825772310153104 ) ) ;
#7156=DIRECTION ( 'NONE',  ( 2.857391495672265093E-16, 4.793132013414519254E-17, 1.000000000000000000 ) ) ;
#7159=CARTESIAN_POINT ( 'NONE',  ( -6.308476396955129850, -59.14191327212131455, -0.5142043607924547954 ) ) ;
#7160=CARTESIAN_POINT ( 'NONE',  ( -1.318626809553760104, -67.28799943462540512, -1.163043645407473958 ) ) ;
#7167=DIRECTION ( 'NONE',  ( 2.290931512739800066E-16, 1.403768413105889815E-16, 1.000000000000000000 ) ) ;
#7169=CARTESIAN_POINT ( 'NONE',  ( 3.016248221826935083, -64.97666327952782694, -3.135076956698916728 ) ) ;
#7171=CARTESIAN_POINT ( 'NONE',  ( -1.956775878777010869, -54.45555501790917674, -0.1654709460969512602 ) ) ;
#7173=ORIENTED_EDGE ( 'NONE', *, *, #3346, .T. ) ;
#7180=CARTESIAN_POINT ( 'NONE',  ( 3.660823140336725068, -65.74644859602665292, -1.309095517728299907 ) ) ;
#7181=VERTEX_POINT ( 'NONE', #4217 ) ;
#7185=CARTESIAN_POINT ( 'NONE',  ( 5.164426235684419275, -63.32698789961681030, 0.7537993011490951023 ) ) ;
#7188=CARTESIAN_POINT ( 'NONE',  ( 5.766935121390225127, -60.94769942240537119, -1.455549280073787921 ) ) ;
#7190=EDGE_CURVE ( 'NONE', #7181, #4852, #3997, .T. ) ;
#7195=CARTESIAN_POINT ( 'NONE',  ( -14.04303360023105895, -37.12711394412414734, 0.03124720627272013079 ) ) ;
#7197=CARTESIAN_POINT ( 'NONE',  ( 6.144163068047750365, -64.45449589790229084, 2.063594979539779661 ) ) ;
#7206=CARTESIAN_POINT ( 'NONE',  ( -1.607783425601855054, -65.25734987882880489, 1.942476202525789342 ) ) ;
#7208=CARTESIAN_POINT ( 'NONE',  ( -3.636793936007903572, -65.52149246903836399, 1.198211322333656348 ) ) ;
#7213=SHAPE_DEFINITION_REPRESENTATION ( #6568, #7047 ) ;
#7215=DIRECTION ( 'NONE',  ( 0.3128463504745289669, 0.9445772445362837777, 0.09950371902099817978 ) ) ;
#7218=CARTESIAN_POINT ( 'NONE',  ( 2.241808083868705115, -67.04438815209937275, -1.340794555410016020 ) ) ;
#7221=ORIENTED_EDGE ( 'NONE', *, *, #4240, .F. ) ;
#7223=CARTESIAN_POINT ( 'NONE',  ( -9.311346830843410416, -51.41373841511902043, 2.533728595105000370 ) ) ;
#7224=CARTESIAN_POINT ( 'NONE',  ( 6.265638173095489982, -61.94185186372677521, 0.5461908750427398873 ) ) ;
#7232=CARTESIAN_POINT ( 'NONE',  ( 7.003919171491410189, -62.62977488282763261, 1.976316849587809843 ) ) ;
#7235=AXIS2_PLACEMENT_3D ( 'NONE', #1645, #4869, #6039 ) ;
#7237=ORIENTED_EDGE ( 'NONE', *, *, #2334, .T. ) ;
#7243=CARTESIAN_POINT ( 'NONE',  ( -4.663084970140659813, -61.97199652813008441, 2.252239320826900482 ) ) ;
#7245=EDGE_CURVE ( 'NONE', #6077, #1508, #522, .T. ) ;
#7246=CARTESIAN_POINT ( 'NONE',  ( 1.018343067164889204, -66.66658444643495329, 0.9358771171724069582 ) ) ;
#7247=EDGE_CURVE ( 'NONE', #6757, #2618, #1360, .T. ) ;
#7251=ORIENTED_EDGE ( 'NONE', *, *, #7152, .T. ) ;
#7252=AXIS2_PLACEMENT_3D ( 'NONE', #589, #3413, #2915 ) ;
#7258=CARTESIAN_POINT ( 'NONE',  ( 5.619938529503549773, -63.59344562873818774, 0.6343307546824898946 ) ) ;
#7259=CIRCLE ( 'NONE', #2690, 0.4999999999999995559 ) ;
#7262=CARTESIAN_POINT ( 'NONE',  ( 1.402950248545461909, -54.15620739517822813, 0.01614447287717020105 ) ) ;
#7269=CARTESIAN_POINT ( 'NONE',  ( 6.577191010720946807, -62.60348822714410488, -2.056697675161959893 ) ) ;
#7270=CARTESIAN_POINT ( 'NONE',  ( 2.241808083868705115, -67.04438815209937275, -1.340794555410016020 ) ) ;
#7272=VERTEX_POINT ( 'NONE', #3826 ) ;
#7277=CARTESIAN_POINT ( 'NONE',  ( 4.837585924071849952, -61.97584320105620748, 1.412225657785534327 ) ) ;
#7279=CARTESIAN_POINT ( 'NONE',  ( -5.060928412568097556, -56.78184410889874556, -0.3751579969454835739 ) ) ;
#7281=EDGE_LOOP ( 'NONE', ( #1367, #3807, #6321, #1080, #5616, #6055 ) ) ;
#7286=EDGE_CURVE ( 'NONE', #2328, #210, #5700, .T. ) ;
#7288=DIRECTION ( 'NONE',  ( -0.2467992669038191755, 0.02032136184815236737, 0.9688535307818070264 ) ) ;
#7290=CARTESIAN_POINT ( 'NONE',  ( -7.175161506198990402, -58.91160695923000645, -1.204451995733903935 ) ) ;
#7296=CARTESIAN_POINT ( 'NONE',  ( -1.592557218785495055, -66.68601476236933934, 1.076257986235874764 ) ) ;
#7305=CARTESIAN_POINT ( 'NONE',  ( -3.328771606340945155, -66.98264282425255089, -1.647280098378362867 ) ) ;
#7309=CARTESIAN_POINT ( 'NONE',  ( 2.467202665543605011, -65.15865635802147438, 2.695445654378740397 ) ) ;
#7312=CARTESIAN_POINT ( 'NONE',  ( 4.653184118170510253, -62.00177009570858644, -2.783824188434504521 ) ) ;
#7315=EDGE_LOOP ( 'NONE', ( #1507, #1784, #5724, #6246, #1483, #1699 ) ) ;
#7318=VERTEX_POINT ( 'NONE', #5046 ) ;
#7322=DIRECTION ( 'NONE',  ( 0.3144066910790611624, 0.9492883822130743221, 0.000000000000000000 ) ) ;
#7325=CARTESIAN_POINT ( 'NONE',  ( 6.472013764049630247, -56.98767972836586182, 1.711274884184114775 ) ) ;
#7326=AXIS2_PLACEMENT_3D ( 'NONE', #6707, #3803, #4385 ) ;
#7328=EDGE_CURVE ( 'NONE', #4770, #1906, #4938, .T. ) ;
#7330=DIRECTION ( 'NONE',  ( -0.2163384215910431896, -0.07165063022625259292, 0.9736857165079894072 ) ) ;
#7331=CARTESIAN_POINT ( 'NONE',  ( 3.403992074353090036, -54.97443010399496899, 2.224669212202579960 ) ) ;
#7332=TOROIDAL_SURFACE ( 'NONE', #3840, 1.500000000000000000, 1.000000000000000000 ) ;
#7333=MANIFOLD_SOLID_BREP ( 'NONE', #2056 ) ;
#7342=CARTESIAN_POINT ( 'NONE',  ( 1.647567807763375081, -53.54661630431167652, -1.692287459705078101 ) ) ;
#7345=DIRECTION ( 'NONE',  ( -0.5224671166576538850, 0.8526594349512809368, 0.000000000000000000 ) ) ;
#7346=CARTESIAN_POINT ( 'NONE',  ( 4.653184118170510253, -62.00177009570858644, -2.783824188434504521 ) ) ;
#7348=DIRECTION ( 'NONE',  ( -0.3144019573014849023, 0.9492899500389726519, 0.000000000000000000 ) ) ;
#7350=CARTESIAN_POINT ( 'NONE',  ( 2.818173014649640429, -55.92969527921476924, 1.989760685886134972 ) ) ;
#7353=CARTESIAN_POINT ( 'NONE',  ( -5.984900349171567768, -62.40475500745689175, -0.6898787680826136137 ) ) ;
#7357=AXIS2_PLACEMENT_3D ( 'NONE', #4150, #7041, #6938 ) ;
#7358=AXIS2_PLACEMENT_3D ( 'NONE', #2368, #3949, #597 ) ;
#7364=CARTESIAN_POINT ( 'NONE',  ( 5.975049724055580214, -64.37929422792591083, -2.133092136665421190 ) ) ;
#7366=VECTOR ( 'NONE', #6836, 1000.000000000000114 ) ;
#7367=ORIENTED_EDGE ( 'NONE', *, *, #2113, .T. ) ;
#7368=AXIS2_PLACEMENT_3D ( 'NONE', #1455, #188, #6579 ) ;
#7370=SURFACE_STYLE_FILL_AREA ( #6887 ) ;
#7372=CARTESIAN_POINT ( 'NONE',  ( 6.187144687173720570, -58.64655194120005177, 0.3691021985165400809 ) ) ;
#7382=EDGE_CURVE ( 'NONE', #1758, #1972, #1941, .T. ) ;
#7386=CARTESIAN_POINT ( 'NONE',  ( 5.904685685680689744, -64.36828453093134783, 1.045689304822035037 ) ) ;
#7390=CARTESIAN_POINT ( 'NONE',  ( 2.735691016399460107, -56.17047939608508500, 0.9718516700694501687 ) ) ;
#7394=CARTESIAN_POINT ( 'NONE',  ( 4.890810490072590611, -59.09042288871975757, -0.8837144134564199893 ) ) ;
#7397=CARTESIAN_POINT ( 'NONE',  ( 2.440761905804889942, -65.30842328614467363, 1.105894752426585415 ) ) ;
#7405=CARTESIAN_POINT ( 'NONE',  ( -7.067610632470020526, -58.47094543896879060, 0.9162228916581999227 ) ) ;
#7409=DIRECTION ( 'NONE',  ( -0.9492883822130750993, 0.3144066910790586089, 0.000000000000000000 ) ) ;
#7420=CARTESIAN_POINT ( 'NONE',  ( -6.733769393910259637, -61.90091566649680743, 1.831080987178660191 ) ) ;
#7428=CARTESIAN_POINT ( 'NONE',  ( 5.191094514348209898, -57.61090315545595786, 2.520404771314449732 ) ) ;
#7440=CARTESIAN_POINT ( 'NONE',  ( 3.193531232915834739, -66.77446787883670254, 1.223174286645849929 ) ) ;
ENDSEC;
END-ISO-10303-21;
